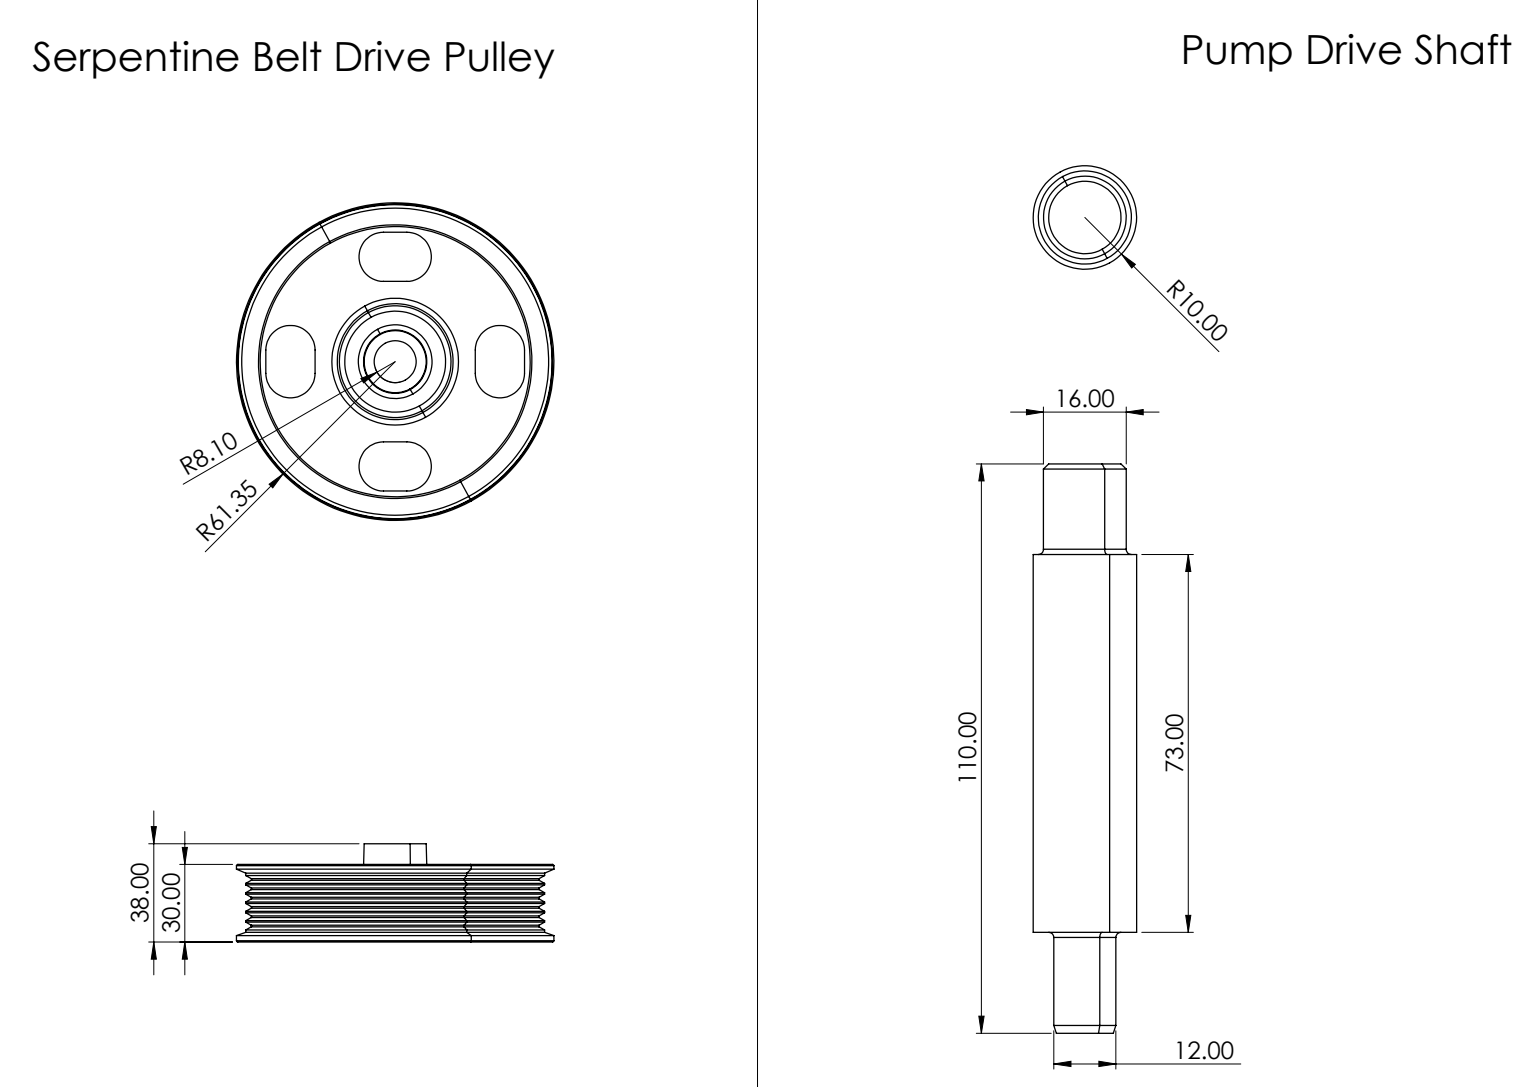
ISO-10303-21;
HEADER;
FILE_DESCRIPTION (('STEP AP214'),
    '1' );
FILE_NAME ('Serpentine Belt Drive Pulley.step',
    '2026-10-09T13:19:41',
    ( '' ),
    ( '' ),
    'SwSTEP 2.0',
    'SolidWorks 2026',
    '' );
FILE_SCHEMA (( 'AUTOMOTIVE_DESIGN' ));
ENDSEC;

DATA;
#8=CARTESIAN_POINT ( 'NONE',  ( 11.78548194719999920, -15.31994771319999948, 21.57317999869999881 ) ) ;
#14=CARTESIAN_POINT ( 'NONE',  ( 0.000000000000000000, -31.69999999999999929, 0.000000000000000000 ) ) ;
#18=CIRCLE ( 'NONE', #19870, 0.3500000000000003664 ) ;
#20=ORIENTED_EDGE ( 'NONE', *, *, #20137, .T. ) ;
#22=VERTEX_POINT ( 'NONE', #6246 ) ;
#29=DIRECTION ( 'NONE',  ( 0.000000000000000000, -1.000000000000000000, 0.000000000000000000 ) ) ;
#31=DIRECTION ( 'NONE',  ( 0.4794255386042040601, 0.000000000000000000, 0.8775825618903720926 ) ) ;
#44=CONICAL_SURFACE ( 'NONE', #19544, 55.67692378859999280, 1.047197551199999799 ) ;
#54=VERTEX_POINT ( 'NONE', #28244 ) ;
#64=CIRCLE ( 'NONE', #16341, 0.3500000000000003664 ) ;
#76=DIRECTION ( 'NONE',  ( 0.4794255386042042266, 0.000000000000000000, 0.8775825618903720926 ) ) ;
#77=VERTEX_POINT ( 'NONE', #6989 ) ;
#84=DIRECTION ( 'NONE',  ( 1.000000000000000000, 0.000000000000000000, 0.000000000000000000 ) ) ;
#87=VERTEX_POINT ( 'NONE', #24762 ) ;
#100=CIRCLE ( 'NONE', #13575, 52.20000000000000284 ) ;
#103=VERTEX_POINT ( 'NONE', #2623 ) ;
#125=ADVANCED_FACE ( 'NONE', ( #15853 ), #9081, .F. ) ;
#128=ORIENTED_EDGE ( 'NONE', *, *, #22826, .F. ) ;
#143=AXIS2_PLACEMENT_3D ( 'NONE', #11532, #26560, #20442 ) ;
#152=DIRECTION ( 'NONE',  ( 0.4794255386042040601, 0.000000000000000000, 0.8775825618903720926 ) ) ;
#157=EDGE_CURVE ( 'NONE', #20862, #20652, #26784, .T. ) ;
#162=DIRECTION ( 'NONE',  ( 0.000000000000000000, 1.000000000000000000, 0.000000000000000000 ) ) ;
#165=ADVANCED_FACE ( 'NONE', ( #26356 ), #6385, .F. ) ;
#169=DIRECTION ( 'NONE',  ( 0.000000000000000000, 1.000000000000000000, 0.000000000000000000 ) ) ;
#171=CARTESIAN_POINT ( 'NONE',  ( 0.000000000000000000, -37.50000000000000000, 0.000000000000000000 ) ) ;
#172=ORIENTED_EDGE ( 'NONE', *, *, #20476, .T. ) ;
#174=DIRECTION ( 'NONE',  ( 0.4794255386042042266, 0.000000000000000000, 0.8775825618903720926 ) ) ;
#177=DIRECTION ( 'NONE',  ( 0.000000000000000000, 1.000000000000000000, 0.000000000000000000 ) ) ;
#188=DIRECTION ( 'NONE',  ( 0.4794255386042000078, 0.000000000000000000, 0.8775825618903743131 ) ) ;
#190=ORIENTED_EDGE ( 'NONE', *, *, #2721, .F. ) ;
#193=CARTESIAN_POINT ( 'NONE',  ( 0.000000000000000000, -23.00000000000000000, 0.000000000000000000 ) ) ;
#207=AXIS2_PLACEMENT_3D ( 'NONE', #10252, #6026, #27775 ) ;
#218=FACE_OUTER_BOUND ( 'NONE', #16317, .T. ) ;
#231=CYLINDRICAL_SURFACE ( 'NONE', #19067, 8.099999999999997868 ) ;
#245=CIRCLE ( 'NONE', #4394, 58.54999999999999716 ) ;
#250=CIRCLE ( 'NONE', #27231, 57.75000000000000000 ) ;
#255=ADVANCED_FACE ( 'NONE', ( #17790 ), #18406, .F. ) ;
#258=VERTEX_POINT ( 'NONE', #22459 ) ;
#265=CARTESIAN_POINT ( 'NONE',  ( 0.000000000000000000, -26.90310889129999694, 0.000000000000000000 ) ) ;
#268=LINE ( 'NONE', #1996, #17176 ) ;
#307=DIRECTION ( 'NONE',  ( 0.000000000000000000, 1.000000000000000000, 0.000000000000000000 ) ) ;
#316=AXIS2_PLACEMENT_3D ( 'NONE', #22770, #793, #16190 ) ;
#318=CARTESIAN_POINT ( 'NONE',  ( 0.000000000000000000, -11.00000000000000000, 0.000000000000000000 ) ) ;
#352=EDGE_CURVE ( 'NONE', #18033, #14401, #4448, .T. ) ;
#357=EDGE_CURVE ( 'NONE', #20895, #2845, #5405, .T. ) ;
#360=ORIENTED_EDGE ( 'NONE', *, *, #15898, .T. ) ;
#367=AXIS2_PLACEMENT_3D ( 'NONE', #6686, #4637, #15550 ) ;
#368=ADVANCED_FACE ( 'NONE', ( #27069 ), #19745, .T. ) ;
#369=CIRCLE ( 'NONE', #15692, 60.85000000000000142 ) ;
#370=DIRECTION ( 'NONE',  ( 0.000000000000000000, 1.000000000000000000, 0.000000000000000000 ) ) ;
#384=CARTESIAN_POINT ( 'NONE',  ( 3.883346862689999845, -2.000000000000000000, 7.108418751309999450 ) ) ;
#385=AXIS2_PLACEMENT_3D ( 'NONE', #10663, #12718, #21630 ) ;
#398=AXIS2_PLACEMENT_3D ( 'NONE', #25664, #5557, #14574 ) ;
#408=DIRECTION ( 'NONE',  ( 0.000000000000000000, 1.000000000000000000, 0.000000000000000000 ) ) ;
#412=CIRCLE ( 'NONE', #28280, 57.75000000000000000 ) ;
#422=ORIENTED_EDGE ( 'NONE', *, *, #27436, .F. ) ;
#424=CARTESIAN_POINT ( 'NONE',  ( -4.500000000000000000, -11.00000000000000000, 31.00000000000000000 ) ) ;
#429=EDGE_CURVE ( 'NONE', #15620, #8975, #245, .T. ) ;
#432=DIRECTION ( 'NONE',  ( -1.000000000000000000, 0.000000000000000000, -4.565061778886334044E-16 ) ) ;
#433=DIRECTION ( 'NONE',  ( 0.4151946956541399669, 0.5000000000001689759, 0.7600087925152558821 ) ) ;
#436=DIRECTION ( 'NONE',  ( -1.224606353819999829E-16, 0.000000000000000000, 1.000000000000000000 ) ) ;
#454=CONICAL_SURFACE ( 'NONE', #1820, 55.67692378859999280, 1.047197551199999799 ) ;
#456=EDGE_CURVE ( 'NONE', #25924, #731, #15538, .T. ) ;
#459=CARTESIAN_POINT ( 'NONE',  ( 27.68682485439999752, -17.30000000000000071, 50.68039294919999804 ) ) ;
#463=DIRECTION ( 'NONE',  ( 0.000000000000000000, 1.000000000000000000, 0.000000000000000000 ) ) ;
#467=ADVANCED_FACE ( 'NONE', ( #20064 ), #15828, .T. ) ;
#474=DIRECTION ( 'NONE',  ( 0.000000000000000000, 1.000000000000000000, 0.000000000000000000 ) ) ;
#476=EDGE_LOOP ( 'NONE', ( #14422, #15237, #5808, #25954 ) ) ;
#481=DIRECTION ( 'NONE',  ( 0.000000000000000000, 1.000000000000000000, 0.000000000000000000 ) ) ;
#484=ORIENTED_EDGE ( 'NONE', *, *, #2417, .F. ) ;
#490=DIRECTION ( 'NONE',  ( 0.4794255386042036715, 0.000000000000000000, 0.8775825618903724257 ) ) ;
#503=EDGE_CURVE ( 'NONE', #1478, #12804, #17430, .T. ) ;
#509=EDGE_LOOP ( 'NONE', ( #14292, #25818, #23874, #1797 ) ) ;
#513=FACE_OUTER_BOUND ( 'NONE', #18198, .T. ) ;
#519=VERTEX_POINT ( 'NONE', #424 ) ;
#526=CARTESIAN_POINT ( 'NONE',  ( 5.873292863139999653, -11.55246854740000018, 10.75099047199999980 ) ) ;
#530=FACE_OUTER_BOUND ( 'NONE', #1949, .T. ) ;
#546=CARTESIAN_POINT ( 'NONE',  ( 27.68682485439999752, -14.30000000000000071, 50.68039294919999804 ) ) ;
#550=ORIENTED_EDGE ( 'NONE', *, *, #21053, .T. ) ;
#575=DIRECTION ( 'NONE',  ( 0.4794255386042000078, 0.000000000000000000, 0.8775825618903743131 ) ) ;
#577=VECTOR ( 'NONE', #18094, 1000.000000000000000 ) ;
#579=VECTOR ( 'NONE', #5626, 999.9999999999998863 ) ;
#581=CARTESIAN_POINT ( 'NONE',  ( 0.000000000000000000, -37.08699221940000257, 0.000000000000000000 ) ) ;
#584=VERTEX_POINT ( 'NONE', #13793 ) ;
#594=ORIENTED_EDGE ( 'NONE', *, *, #7560, .T. ) ;
#599=ORIENTED_EDGE ( 'NONE', *, *, #25882, .T. ) ;
#604=ORIENTED_EDGE ( 'NONE', *, *, #24072, .T. ) ;
#618=VERTEX_POINT ( 'NONE', #23274 ) ;
#636=ORIENTED_EDGE ( 'NONE', *, *, #17902, .T. ) ;
#640=VERTEX_POINT ( 'NONE', #18620 ) ;
#669=EDGE_CURVE ( 'NONE', #15395, #12657, #1152, .T. ) ;
#673=EDGE_CURVE ( 'NONE', #12096, #23467, #9990, .T. ) ;
#691=CIRCLE ( 'NONE', #4371, 24.76278252470000041 ) ;
#703=DIRECTION ( 'NONE',  ( 0.000000000000000000, 1.000000000000000000, 0.000000000000000000 ) ) ;
#704=TOROIDAL_SURFACE ( 'NONE', #18826, 25.11294200180000047, 0.5000000000000000000 ) ;
#721=LINE ( 'NONE', #9422, #6410 ) ;
#731=VERTEX_POINT ( 'NONE', #1559 ) ;
#736=CIRCLE ( 'NONE', #10888, 0.3500000000000003664 ) ;
#739=AXIS2_PLACEMENT_3D ( 'NONE', #22838, #3037, #27350 ) ;
#764=ORIENTED_EDGE ( 'NONE', *, *, #15472, .F. ) ;
#765=CARTESIAN_POINT ( 'NONE',  ( 25.57735248450000043, -16.00000000000000000, 46.81902967690000139 ) ) ;
#770=ORIENTED_EDGE ( 'NONE', *, *, #5118, .F. ) ;
#786=CIRCLE ( 'NONE', #28633, 0.3500000000000003664 ) ;
#793=DIRECTION ( 'NONE',  ( 0.000000000000000000, 1.000000000000000000, 0.000000000000000000 ) ) ;
#803=VECTOR ( 'NONE', #16768, 999.9999999999998863 ) ;
#810=DIRECTION ( 'NONE',  ( 1.000000000000000000, 0.000000000000000000, 0.000000000000000000 ) ) ;
#852=ORIENTED_EDGE ( 'NONE', *, *, #4107, .F. ) ;
#859=CIRCLE ( 'NONE', #18511, 57.75000000000000000 ) ;
#863=CARTESIAN_POINT ( 'NONE',  ( 4.500000000000000000, -13.00000000000000000, -50.00000000000000000 ) ) ;
#872=DIRECTION ( 'NONE',  ( 0.000000000000000000, 0.000000000000000000, -1.000000000000000000 ) ) ;
#900=CIRCLE ( 'NONE', #15733, 53.35000000000000142 ) ;
#914=VERTEX_POINT ( 'NONE', #15022 ) ;
#940=AXIS2_PLACEMENT_3D ( 'NONE', #13156, #4429, #22204 ) ;
#943=ADVANCED_FACE ( 'NONE', ( #22484 ), #23059, .T. ) ;
#954=CARTESIAN_POINT ( 'NONE',  ( 0.000000000000000000, -10.00000000000000000, 60.66666666670000296 ) ) ;
#963=DIRECTION ( 'NONE',  ( 0.3422283636740854340, 0.7003189540771749266, 0.6264448177271558782 ) ) ;
#975=ORIENTED_EDGE ( 'NONE', *, *, #2781, .F. ) ;
#984=AXIS2_PLACEMENT_3D ( 'NONE', #22104, #28780, #24280 ) ;
#999=FACE_OUTER_BOUND ( 'NONE', #16209, .T. ) ;
#1007=LINE ( 'NONE', #25323, #579 ) ;
#1009=ORIENTED_EDGE ( 'NONE', *, *, #8094, .T. ) ;
#1033=CARTESIAN_POINT ( 'NONE',  ( 0.000000000000000000, -2.000000000000000000, 0.000000000000000000 ) ) ;
#1048=TOROIDAL_SURFACE ( 'NONE', #18699, 57.54999999999999716, 1.000000000000000000 ) ;
#1057=ORIENTED_EDGE ( 'NONE', *, *, #2655, .F. ) ;
#1060=CIRCLE ( 'NONE', #4744, 14.25000000000000000 ) ;
#1067=ORIENTED_EDGE ( 'NONE', *, *, #7433, .T. ) ;
#1075=ORIENTED_EDGE ( 'NONE', *, *, #3374, .F. ) ;
#1104=AXIS2_PLACEMENT_3D ( 'NONE', #1320, #19082, #16896 ) ;
#1110=DIRECTION ( 'NONE',  ( 0.000000000000000000, -1.000000000000000000, 0.000000000000000000 ) ) ;
#1114=CARTESIAN_POINT ( 'NONE',  ( 0.000000000000000000, -15.14308496720000008, 0.000000000000000000 ) ) ;
#1122=CONICAL_SURFACE ( 'NONE', #9854, 11.99999999999999822, 0.02623728384790100648 ) ;
#1131=CYLINDRICAL_SURFACE ( 'NONE', #24779, 61.34999999999998721 ) ;
#1132=ORIENTED_EDGE ( 'NONE', *, *, #23898, .T. ) ;
#1134=ADVANCED_FACE ( 'NONE', ( #21028 ), #16056, .T. ) ;
#1142=CARTESIAN_POINT ( 'NONE',  ( 0.000000000000000000, -2.000000000000000000, 0.000000000000000000 ) ) ;
#1145=DIRECTION ( 'NONE',  ( 1.000000000000000000, 0.000000000000000000, 0.000000000000000000 ) ) ;
#1150=CONICAL_SURFACE ( 'NONE', #12714, 21.60095686220001454, 0.7949521073230001456 ) ;
#1152=LINE ( 'NONE', #7700, #5344 ) ;
#1170=ORIENTED_EDGE ( 'NONE', *, *, #26606, .F. ) ;
#1174=CARTESIAN_POINT ( 'NONE',  ( 0.000000000000000000, -17.50000000000000000, 9.099999999999999645 ) ) ;
#1180=DIRECTION ( 'NONE',  ( 1.000000000000000000, 0.000000000000000000, 0.000000000000000000 ) ) ;
#1181=VERTEX_POINT ( 'NONE', #28133 ) ;
#1186=EDGE_CURVE ( 'NONE', #5075, #17731, #27244, .T. ) ;
#1194=EDGE_LOOP ( 'NONE', ( #8651, #2603, #6295, #28164 ) ) ;
#1196=EDGE_CURVE ( 'NONE', #14426, #19773, #20727, .T. ) ;
#1201=ORIENTED_EDGE ( 'NONE', *, *, #3911, .F. ) ;
#1212=FACE_OUTER_BOUND ( 'NONE', #25199, .T. ) ;
#1222=EDGE_CURVE ( 'NONE', #14011, #25949, #25369, .T. ) ;
#1223=DIRECTION ( 'NONE',  ( 1.000000000000000000, 0.000000000000000000, 0.000000000000000000 ) ) ;
#1228=CARTESIAN_POINT ( 'NONE',  ( 0.000000000000000000, -36.20000000000000284, 0.000000000000000000 ) ) ;
#1234=VERTEX_POINT ( 'NONE', #26969 ) ;
#1239=DIRECTION ( 'NONE',  ( 0.4794255386042000078, 0.000000000000000000, 0.8775825618903743131 ) ) ;
#1252=DIRECTION ( 'NONE',  ( 0.4794255386042040601, 0.000000000000000000, 0.8775825618903720926 ) ) ;
#1258=CARTESIAN_POINT ( 'NONE',  ( -4.500000000000000000, -15.00000000000000000, 40.50000000000000000 ) ) ;
#1269=DIRECTION ( 'NONE',  ( 1.000000000000000000, 0.000000000000000000, 0.000000000000000000 ) ) ;
#1274=ORIENTED_EDGE ( 'NONE', *, *, #6243, .T. ) ;
#1286=DIRECTION ( 'NONE',  ( -1.000000000000000000, 0.000000000000000000, 0.000000000000000000 ) ) ;
#1299=CIRCLE ( 'NONE', #22695, 52.86371681420000357 ) ;
#1320=CARTESIAN_POINT ( 'NONE',  ( 0.000000000000000000, -2.000000000000000000, 8.099999999999999645 ) ) ;
#1323=AXIS2_PLACEMENT_3D ( 'NONE', #7852, #12345, #17150 ) ;
#1336=EDGE_LOOP ( 'NONE', ( #27422, #1067, #8213, #19531 ) ) ;
#1337=CIRCLE ( 'NONE', #5040, 55.67692378859999991 ) ;
#1338=FACE_OUTER_BOUND ( 'NONE', #23635, .T. ) ;
#1339=AXIS2_PLACEMENT_3D ( 'NONE', #8246, #19612, #25892 ) ;
#1348=CARTESIAN_POINT ( 'NONE',  ( 28.07036528529999941, -39.32601556110000018, 51.38245899869999533 ) ) ;
#1357=ORIENTED_EDGE ( 'NONE', *, *, #15472, .T. ) ;
#1360=DIRECTION ( 'NONE',  ( 0.000000000000000000, -1.000000000000000000, 0.000000000000000000 ) ) ;
#1369=CARTESIAN_POINT ( 'NONE',  ( -31.00000000000000000, 0.000000000000000000, -4.500000000000000000 ) ) ;
#1373=AXIS2_PLACEMENT_3D ( 'NONE', #19047, #27930, #7968 ) ;
#1377=EDGE_CURVE ( 'NONE', #2012, #20039, #5529, .T. ) ;
#1381=EDGE_CURVE ( 'NONE', #22328, #8830, #3355, .T. ) ;
#1383=TOROIDAL_SURFACE ( 'NONE', #5566, 14.25000000000000000, 2.000000000000000000 ) ;
#1386=AXIS2_PLACEMENT_3D ( 'NONE', #5883, #3432, #1535 ) ;
#1392=( LENGTH_UNIT ( ) NAMED_UNIT ( * ) SI_UNIT ( .MILLI., .METRE. ) );
#1394=AXIS2_PLACEMENT_3D ( 'NONE', #27280, #26988, #18533 ) ;
#1401=CIRCLE ( 'NONE', #5114, 61.35000000000000142 ) ;
#1412=EDGE_LOOP ( 'NONE', ( #2757, #20982, #9366, #23861 ) ) ;
#1424=ORIENTED_EDGE ( 'NONE', *, *, #18031, .F. ) ;
#1434=ADVANCED_FACE ( 'NONE', ( #8401 ), #24419, .F. ) ;
#1441=DIRECTION ( 'NONE',  ( 0.000000000000000000, 1.000000000000000000, 0.000000000000000000 ) ) ;
#1449=ORIENTED_EDGE ( 'NONE', *, *, #5830, .T. ) ;
#1451=CIRCLE ( 'NONE', #4700, 0.4999999999999981126 ) ;
#1454=ORIENTED_EDGE ( 'NONE', *, *, #12507, .T. ) ;
#1456=CARTESIAN_POINT ( 'NONE',  ( 31.00000000000000000, -11.00000000000000000, 1.953992523340000041E-14 ) ) ;
#1457=ORIENTED_EDGE ( 'NONE', *, *, #19024, .T. ) ;
#1478=VERTEX_POINT ( 'NONE', #27890 ) ;
#1494=CARTESIAN_POINT ( 'NONE',  ( 0.000000000000000000, -40.00000000000000000, 60.85000000000000142 ) ) ;
#1497=CONICAL_SURFACE ( 'NONE', #22909, 57.74999999999999289, 1.152571997220000144 ) ;
#1519=VECTOR ( 'NONE', #12148, 1000.000000000000000 ) ;
#1535=DIRECTION ( 'NONE',  ( 0.4794255386042040601, 0.000000000000000000, 0.8775825618903720926 ) ) ;
#1536=EDGE_LOOP ( 'NONE', ( #13375, #8343, #24939, #21800 ) ) ;
#1559=CARTESIAN_POINT ( 'NONE',  ( 26.69293917519999937, -22.69689110870000093, 48.86109741659999628 ) ) ;
#1563=DIRECTION ( 'NONE',  ( 0.000000000000000000, -1.000000000000000000, 0.000000000000000000 ) ) ;
#1567=CIRCLE ( 'NONE', #15021, 60.66666666670000296 ) ;
#1595=EDGE_LOOP ( 'NONE', ( #10372, #9875, #25781, #7720 ) ) ;
#1599=EDGE_LOOP ( 'NONE', ( #20525, #22685, #3053, #14488 ) ) ;
#1610=CARTESIAN_POINT ( 'NONE',  ( -27.68682485439999752, -32.30000000000000426, -50.68039294919999804 ) ) ;
#1618=AXIS2_PLACEMENT_3D ( 'NONE', #8826, #2740, #575 ) ;
#1621=CARTESIAN_POINT ( 'NONE',  ( 0.000000000000000000, -33.49689110869999809, 0.000000000000000000 ) ) ;
#1637=FACE_OUTER_BOUND ( 'NONE', #11830, .T. ) ;
#1640=DIRECTION ( 'NONE',  ( 1.000000000000000000, 0.000000000000000000, 0.000000000000000000 ) ) ;
#1649=CIRCLE ( 'NONE', #16987, 0.3500000000000003664 ) ;
#1654=ORIENTED_EDGE ( 'NONE', *, *, #12704, .T. ) ;
#1656=EDGE_CURVE ( 'NONE', #15453, #19773, #6655, .T. ) ;
#1668=EDGE_LOOP ( 'NONE', ( #8051, #17208, #12347, #594 ) ) ;
#1699=CARTESIAN_POINT ( 'NONE',  ( -9.348798002780000616, -17.50000000000000000, -17.11285995690000306 ) ) ;
#1704=CARTESIAN_POINT ( 'NONE',  ( 0.000000000000000000, -11.79999999999999893, 0.000000000000000000 ) ) ;
#1711=DIRECTION ( 'NONE',  ( 1.000000000000000000, 0.000000000000000000, 0.000000000000000000 ) ) ;
#1732=CARTESIAN_POINT ( 'NONE',  ( 0.000000000000000000, -11.00000000000000000, 0.000000000000000000 ) ) ;
#1737=ORIENTED_EDGE ( 'NONE', *, *, #10273, .F. ) ;
#1742=CIRCLE ( 'NONE', #25487, 24.40223267850000255 ) ;
#1746=EDGE_CURVE ( 'NONE', #914, #1181, #8053, .T. ) ;
#1750=DIRECTION ( 'NONE',  ( 0.4794255386042040046, 0.000000000000000000, 0.8775825618903722036 ) ) ;
#1752=DIRECTION ( 'NONE',  ( 0.4794255386042059475, 0.000000000000000000, 0.8775825618903710934 ) ) ;
#1753=EDGE_CURVE ( 'NONE', #8830, #25924, #27612, .T. ) ;
#1757=ORIENTED_EDGE ( 'NONE', *, *, #22845, .T. ) ;
#1760=ORIENTED_EDGE ( 'NONE', *, *, #23659, .T. ) ;
#1766=DIRECTION ( 'NONE',  ( 0.4794255386042040046, 0.000000000000000000, 0.8775825618903720926 ) ) ;
#1768=DIRECTION ( 'NONE',  ( 0.4794255386042000078, 0.000000000000000000, 0.8775825618903743131 ) ) ;
#1769=DIRECTION ( 'NONE',  ( 0.000000000000000000, 1.000000000000000000, 0.000000000000000000 ) ) ;
#1773=VECTOR ( 'NONE', #7996, 1000.000000000000000 ) ;
#1786=( GEOMETRIC_REPRESENTATION_CONTEXT ( 3 ) GLOBAL_UNCERTAINTY_ASSIGNED_CONTEXT ( ( #20546 ) ) GLOBAL_UNIT_ASSIGNED_CONTEXT ( ( #25669, #21288, #14718 ) ) REPRESENTATION_CONTEXT ( 'NONE', 'WORKASPACE' ) );
#1797=ORIENTED_EDGE ( 'NONE', *, *, #15743, .F. ) ;
#1801=CARTESIAN_POINT ( 'NONE',  ( -25.02601311510000315, -11.00000000000000000, -45.80980973070000317 ) ) ;
#1802=ORIENTED_EDGE ( 'NONE', *, *, #26480, .T. ) ;
#1819=AXIS2_PLACEMENT_3D ( 'NONE', #7307, #9621, #5264 ) ;
#1820=AXIS2_PLACEMENT_3D ( 'NONE', #12023, #27649, #7692 ) ;
#1834=AXIS2_PLACEMENT_3D ( 'NONE', #19061, #20420, #490 ) ;
#1840=ADVANCED_FACE ( 'NONE', ( #6565 ), #11765, .T. ) ;
#1843=CARTESIAN_POINT ( 'NONE',  ( -29.08514934200000113, -20.00000000000000000, -53.24000875469999983 ) ) ;
#1846=CYLINDRICAL_SURFACE ( 'NONE', #7110, 57.74999999999999289 ) ;
#1856=VERTEX_POINT ( 'NONE', #10899 ) ;
#1868=CARTESIAN_POINT ( 'NONE',  ( -29.41275679339999982, -25.00000000000000000, -53.83969017199999740 ) ) ;
#1871=VERTEX_POINT ( 'NONE', #26828 ) ;
#1874=ORIENTED_EDGE ( 'NONE', *, *, #16751, .T. ) ;
#1875=EDGE_CURVE ( 'NONE', #1478, #12096, #8721, .T. ) ;
#1900=AXIS2_PLACEMENT_3D ( 'NONE', #27713, #25243, #5270 ) ;
#1914=ORIENTED_EDGE ( 'NONE', *, *, #6174, .F. ) ;
#1929=ORIENTED_EDGE ( 'NONE', *, *, #4004, .F. ) ;
#1930=LINE ( 'NONE', #19682, #6678 ) ;
#1933=ORIENTED_EDGE ( 'NONE', *, *, #10541, .T. ) ;
#1944=VERTEX_POINT ( 'NONE', #26975 ) ;
#1945=DIRECTION ( 'NONE',  ( 0.000000000000000000, 1.000000000000000000, 0.000000000000000000 ) ) ;
#1947=EDGE_CURVE ( 'NONE', #19954, #26186, #16169, .T. ) ;
#1949=EDGE_LOOP ( 'NONE', ( #6217, #17280, #3392, #19503 ) ) ;
#1957=ORIENTED_EDGE ( 'NONE', *, *, #7433, .F. ) ;
#1965=DIRECTION ( 'NONE',  ( 0.000000000000000000, 1.000000000000000000, 0.000000000000000000 ) ) ;
#1976=ORIENTED_EDGE ( 'NONE', *, *, #15304, .F. ) ;
#1985=DIRECTION ( 'NONE',  ( 0.000000000000000000, 1.000000000000000000, 0.000000000000000000 ) ) ;
#1988=ORIENTED_EDGE ( 'NONE', *, *, #18804, .T. ) ;
#1992=DIRECTION ( 'NONE',  ( 1.000000000000000000, 0.000000000000000000, 0.000000000000000000 ) ) ;
#1994=DIRECTION ( 'NONE',  ( 0.000000000000000000, 0.000000000000000000, 1.000000000000000000 ) ) ;
#1996=CARTESIAN_POINT ( 'NONE',  ( 27.18988201479999844, -31.10155444569999617, 49.77074518290000071 ) ) ;
#2002=AXIS2_PLACEMENT_3D ( 'NONE', #16319, #2648, #20557 ) ;
#2005=VECTOR ( 'NONE', #1563, 1000.000000000000000 ) ;
#2012=VERTEX_POINT ( 'NONE', #7159 ) ;
#2023=AXIS2_PLACEMENT_3D ( 'NONE', #12263, #20751, #18979 ) ;
#2026=ORIENTED_EDGE ( 'NONE', *, *, #15396, .F. ) ;
#2033=CARTESIAN_POINT ( 'NONE',  ( -9.348798002780000616, -13.50000000000000000, -17.11285995690000306 ) ) ;
#2039=VERTEX_POINT ( 'NONE', #2791 ) ;
#2041=DIRECTION ( 'NONE',  ( 0.4794255386042036715, 0.000000000000000000, 0.8775825618903724257 ) ) ;
#2042=CARTESIAN_POINT ( 'NONE',  ( 0.000000000000000000, -17.50000000000000000, 0.000000000000000000 ) ) ;
#2050=EDGE_CURVE ( 'NONE', #2986, #9393, #22604, .T. ) ;
#2052=VECTOR ( 'NONE', #28538, 1000.000000000000114 ) ;
#2058=ORIENTED_EDGE ( 'NONE', *, *, #21512, .F. ) ;
#2068=DIRECTION ( 'NONE',  ( 0.4794255386042040601, 0.000000000000000000, 0.8775825618903720926 ) ) ;
#2085=ADVANCED_FACE ( 'NONE', ( #25503 ), #5278, .F. ) ;
#2087=ORIENTED_EDGE ( 'NONE', *, *, #429, .T. ) ;
#2100=DIRECTION ( 'NONE',  ( 0.000000000000000000, 1.000000000000000000, 0.000000000000000000 ) ) ;
#2115=DIRECTION ( 'NONE',  ( 0.000000000000000000, 1.000000000000000000, 0.000000000000000000 ) ) ;
#2118=DIRECTION ( 'NONE',  ( 0.4794255386042041156, 0.000000000000000000, 0.8775825618903722036 ) ) ;
#2134=DIRECTION ( 'NONE',  ( 0.4794255386042040601, 0.000000000000000000, 0.8775825618903720926 ) ) ;
#2137=CIRCLE ( 'NONE', #22635, 52.86371681420000357 ) ;
#2138=PLANE ( 'NONE',  #18692 ) ;
#2150=DIRECTION ( 'NONE',  ( 0.4794255386042036715, 0.000000000000000000, 0.8775825618903724257 ) ) ;
#2153=VERTEX_POINT ( 'NONE', #27966 ) ;
#2154=ADVANCED_FACE ( 'NONE', ( #23872, #16748 ), #8005, .T. ) ;
#2165=ORIENTED_EDGE ( 'NONE', *, *, #16459, .T. ) ;
#2190=CARTESIAN_POINT ( 'NONE',  ( 0.000000000000000000, -14.00000000000000000, 0.000000000000000000 ) ) ;
#2194=DIRECTION ( 'NONE',  ( 0.000000000000000000, 1.000000000000000000, 0.000000000000000000 ) ) ;
#2195=ORIENTED_EDGE ( 'NONE', *, *, #16351, .F. ) ;
#2197=EDGE_CURVE ( 'NONE', #19419, #16942, #10351, .T. ) ;
#2216=DIRECTION ( 'NONE',  ( -0.8775825618903722036, 0.000000000000000000, 0.4794255386042041156 ) ) ;
#2223=CIRCLE ( 'NONE', #14769, 58.54999999999999716 ) ;
#2226=CYLINDRICAL_SURFACE ( 'NONE', #28044, 57.74999999999999289 ) ;
#2240=ADVANCED_FACE ( 'NONE', ( #15238 ), #26346, .T. ) ;
#2241=CARTESIAN_POINT ( 'NONE',  ( 0.000000000000000000, -20.89999999999999858, 0.000000000000000000 ) ) ;
#2252=PRODUCT ( 'Serpentine Belt Drive Pulley', 'Serpentine Belt Drive Pulley', '', ( #8864 ) ) ;
#2256=CARTESIAN_POINT ( 'NONE',  ( 0.000000000000000000, -20.00000000000000000, 0.000000000000000000 ) ) ;
#2258=VERTEX_POINT ( 'NONE', #24299 ) ;
#2260=VECTOR ( 'NONE', #22969, 999.9999999999998863 ) ;
#2275=CARTESIAN_POINT ( 'NONE',  ( 0.000000000000000000, -16.50000000000000000, 0.000000000000000000 ) ) ;
#2280=AXIS2_PLACEMENT_3D ( 'NONE', #3506, #12364, #16326 ) ;
#2282=FACE_OUTER_BOUND ( 'NONE', #10560, .T. ) ;
#2295=CIRCLE ( 'NONE', #13919, 9.500000000000000000 ) ;
#2299=CIRCLE ( 'NONE', #5564, 57.75000000000000000 ) ;
#2330=FACE_OUTER_BOUND ( 'NONE', #5988, .T. ) ;
#2339=EDGE_LOOP ( 'NONE', ( #24017, #18856, #23774, #28014 ) ) ;
#2342=ORIENTED_EDGE ( 'NONE', *, *, #23406, .F. ) ;
#2345=CARTESIAN_POINT ( 'NONE',  ( 2.220446049249999745E-14, -15.00000000000000000, -50.00000000000000000 ) ) ;
#2347=ADVANCED_FACE ( 'NONE', ( #11160 ), #18185, .T. ) ;
#2355=FACE_OUTER_BOUND ( 'NONE', #19327, .T. ) ;
#2359=AXIS2_PLACEMENT_3D ( 'NONE', #13477, #22829, #2870 ) ;
#2364=CIRCLE ( 'NONE', #21427, 57.75000000000000000 ) ;
#2371=EDGE_CURVE ( 'NONE', #6736, #4998, #4926, .T. ) ;
#2377=CARTESIAN_POINT ( 'NONE',  ( -26.69293917519999937, -19.09689110869999951, -48.86109741659999628 ) ) ;
#2383=TOROIDAL_SURFACE ( 'NONE', #10709, 55.85192378860000417, 0.3499999999999999778 ) ;
#2384=CIRCLE ( 'NONE', #27960, 55.67692378859999991 ) ;
#2389=VECTOR ( 'NONE', #15810, 1000.000000000000000 ) ;
#2396=CARTESIAN_POINT ( 'NONE',  ( 0.000000000000000000, -23.00000000000000000, 0.000000000000000000 ) ) ;
#2398=DIRECTION ( 'NONE',  ( 0.000000000000000000, 1.000000000000000000, 0.000000000000000000 ) ) ;
#2412=EDGE_CURVE ( 'NONE', #19945, #16942, #21521, .T. ) ;
#2416=FACE_OUTER_BOUND ( 'NONE', #12610, .T. ) ;
#2417=EDGE_CURVE ( 'NONE', #8384, #18741, #27081, .T. ) ;
#2427=ORIENTED_EDGE ( 'NONE', *, *, #12208, .T. ) ;
#2431=DIRECTION ( 'NONE',  ( 0.4751828347227322613, 0.1327433628319252545, 0.8698163445285104212 ) ) ;
#2434=FACE_OUTER_BOUND ( 'NONE', #10940, .T. ) ;
#2457=ADVANCED_FACE ( 'NONE', ( #3186 ), #1122, .T. ) ;
#2464=CARTESIAN_POINT ( 'NONE',  ( 31.00000000000000000, 0.000000000000000000, 4.500000000000000000 ) ) ;
#2487=DIRECTION ( 'NONE',  ( 0.4794255386042040601, 0.000000000000000000, 0.8775825618903720926 ) ) ;
#2490=CIRCLE ( 'NONE', #13571, 61.35000000000000142 ) ;
#2491=AXIS2_PLACEMENT_3D ( 'NONE', #18706, #27860, #8044 ) ;
#2498=ORIENTED_EDGE ( 'NONE', *, *, #27253, .T. ) ;
#2506=EDGE_LOOP ( 'NONE', ( #7714, #6725, #4166, #19968 ) ) ;
#2520=CARTESIAN_POINT ( 'NONE',  ( 0.000000000000000000, -10.50000000000000000, 0.000000000000000000 ) ) ;
#2528=EDGE_CURVE ( 'NONE', #11029, #12945, #19681, .T. ) ;
#2557=PLANE ( 'NONE',  #24883 ) ;
#2560=DIRECTION ( 'NONE',  ( 0.000000000000000000, 1.000000000000000000, 0.000000000000000000 ) ) ;
#2565=CARTESIAN_POINT ( 'NONE',  ( 0.000000000000000000, -20.89999999999999858, 0.000000000000000000 ) ) ;
#2573=ORIENTED_EDGE ( 'NONE', *, *, #17303, .T. ) ;
#2577=EDGE_LOOP ( 'NONE', ( #9350, #10710, #7557, #28137 ) ) ;
#2580=CYLINDRICAL_SURFACE ( 'NONE', #13699, 9.500000000000001776 ) ;
#2590=ORIENTED_EDGE ( 'NONE', *, *, #6883, .T. ) ;
#2599=ORIENTED_EDGE ( 'NONE', *, *, #20782, .F. ) ;
#2603=ORIENTED_EDGE ( 'NONE', *, *, #23973, .T. ) ;
#2609=ORIENTED_EDGE ( 'NONE', *, *, #6058, .F. ) ;
#2623=CARTESIAN_POINT ( 'NONE',  ( -27.68682485439999752, -14.30000000000000071, -50.68039294919999804 ) ) ;
#2625=EDGE_CURVE ( 'NONE', #7539, #5596, #14520, .T. ) ;
#2629=EDGE_CURVE ( 'NONE', #8365, #14272, #16715, .T. ) ;
#2635=ORIENTED_EDGE ( 'NONE', *, *, #22928, .T. ) ;
#2648=DIRECTION ( 'NONE',  ( 0.000000000000000000, 1.000000000000000000, 0.000000000000000000 ) ) ;
#2655=EDGE_CURVE ( 'NONE', #15179, #8526, #2490, .T. ) ;
#2671=DIRECTION ( 'NONE',  ( 0.4794255386042041156, 0.000000000000000000, 0.8775825618903720926 ) ) ;
#2696=AXIS2_PLACEMENT_3D ( 'NONE', #17695, #28613, #4289 ) ;
#2708=DIRECTION ( 'NONE',  ( 0.000000000000000000, 1.000000000000000000, 0.000000000000000000 ) ) ;
#2712=CARTESIAN_POINT ( 'NONE',  ( 27.68682485439999752, -24.80000000000000071, 50.68039294919999804 ) ) ;
#2714=ORIENTED_EDGE ( 'NONE', *, *, #18312, .T. ) ;
#2716=AXIS2_PLACEMENT_3D ( 'NONE', #4651, #13234, #17479 ) ;
#2718=EDGE_LOOP ( 'NONE', ( #27894, #16569, #23075, #22728 ) ) ;
#2721=EDGE_CURVE ( 'NONE', #21247, #17262, #18248, .T. ) ;
#2723=CARTESIAN_POINT ( 'NONE',  ( 0.000000000000000000, -30.20000000000000284, 0.000000000000000000 ) ) ;
#2730=CIRCLE ( 'NONE', #20874, 2.999999999999999556 ) ;
#2740=DIRECTION ( 'NONE',  ( 0.8775825618903722036, 0.000000000000000000, -0.4794255386042041156 ) ) ;
#2746=ORIENTED_EDGE ( 'NONE', *, *, #8123, .T. ) ;
#2748=CARTESIAN_POINT ( 'NONE',  ( 27.18988201479999844, -25.69844555429999744, 49.77074518290000071 ) ) ;
#2750=ORIENTED_EDGE ( 'NONE', *, *, #10665, .T. ) ;
#2753=DIRECTION ( 'NONE',  ( 1.000000000000000000, 0.000000000000000000, 0.000000000000000000 ) ) ;
#2757=ORIENTED_EDGE ( 'NONE', *, *, #18056, .F. ) ;
#2774=CYLINDRICAL_SURFACE ( 'NONE', #25788, 57.74999999999999289 ) ;
#2775=EDGE_LOOP ( 'NONE', ( #20148, #24485, #15477, #18761 ) ) ;
#2780=DIRECTION ( 'NONE',  ( 0.000000000000000000, 1.000000000000000000, 0.000000000000000000 ) ) ;
#2781=EDGE_CURVE ( 'NONE', #731, #6736, #12177, .T. ) ;
#2783=DIRECTION ( 'NONE',  ( 0.000000000000000000, 1.000000000000000000, 0.000000000000000000 ) ) ;
#2784=DIRECTION ( 'NONE',  ( -0.4509255599460827435, -0.3396444637780623443, -0.8254137008871517134 ) ) ;
#2791=CARTESIAN_POINT ( 'NONE',  ( -26.69293917519999937, -15.49689110870000164, -48.86109741659999628 ) ) ;
#2806=DIRECTION ( 'NONE',  ( 1.000000000000000000, 0.000000000000000000, 0.000000000000000000 ) ) ;
#2813=FACE_OUTER_BOUND ( 'NONE', #11451, .T. ) ;
#2816=ADVANCED_FACE ( 'NONE', ( #6344 ), #1846, .T. ) ;
#2826=CARTESIAN_POINT ( 'NONE',  ( 4.500000000000000000, -11.00000000000000000, 31.00000000000000000 ) ) ;
#2845=VERTEX_POINT ( 'NONE', #6494 ) ;
#2858=CARTESIAN_POINT ( 'NONE',  ( 0.000000000000000000, -37.08699221940000257, 0.000000000000000000 ) ) ;
#2861=DIRECTION ( 'NONE',  ( 0.000000000000000000, -1.000000000000000000, 0.000000000000000000 ) ) ;
#2863=ORIENTED_EDGE ( 'NONE', *, *, #21763, .T. ) ;
#2870=DIRECTION ( 'NONE',  ( 0.4794255386042042266, 0.000000000000000000, 0.8775825618903720926 ) ) ;
#2880=VERTEX_POINT ( 'NONE', #25156 ) ;
#2887=ORIENTED_EDGE ( 'NONE', *, *, #24848, .F. ) ;
#2907=EDGE_LOOP ( 'NONE', ( #13611, #23142, #26239, #26486 ) ) ;
#2948=DIRECTION ( 'NONE',  ( 1.000000000000000000, 0.000000000000000000, 0.000000000000000000 ) ) ;
#2960=CYLINDRICAL_SURFACE ( 'NONE', #316, 53.34999999999998721 ) ;
#2975=DIRECTION ( 'NONE',  ( 0.8775825618903722036, 0.000000000000000000, -0.4794255386042041156 ) ) ;
#2986=VERTEX_POINT ( 'NONE', #23391 ) ;
#2992=ADVANCED_FACE ( 'NONE', ( #16679 ), #1131, .T. ) ;
#2995=CIRCLE ( 'NONE', #8084, 55.67692378859999991 ) ;
#3001=ORIENTED_EDGE ( 'NONE', *, *, #15191, .T. ) ;
#3015=ORIENTED_EDGE ( 'NONE', *, *, #26696, .T. ) ;
#3016=CONICAL_SURFACE ( 'NONE', #18352, 55.67692378859999280, 1.047197551199999799 ) ;
#3022=ORIENTED_EDGE ( 'NONE', *, *, #4676, .F. ) ;
#3025=DIRECTION ( 'NONE',  ( 0.000000000000000000, 1.000000000000000000, 0.000000000000000000 ) ) ;
#3027=ADVANCED_FACE ( 'NONE', ( #16547 ), #3570, .T. ) ;
#3028=VECTOR ( 'NONE', #9528, 999.9999999999998863 ) ;
#3035=CARTESIAN_POINT ( 'NONE',  ( 0.000000000000000000, -2.000000000000000000, 0.000000000000000000 ) ) ;
#3037=DIRECTION ( 'NONE',  ( 0.000000000000000000, 1.000000000000000000, 0.000000000000000000 ) ) ;
#3053=ORIENTED_EDGE ( 'NONE', *, *, #27993, .T. ) ;
#3055=DIRECTION ( 'NONE',  ( 0.4794255386042037270, 0.000000000000000000, 0.8775825618903724257 ) ) ;
#3058=CONICAL_SURFACE ( 'NONE', #9988, 8.099999999999997868, 0.7853981633970000820 ) ;
#3071=ORIENTED_EDGE ( 'NONE', *, *, #21876, .F. ) ;
#3078=DIRECTION ( 'NONE',  ( 0.000000000000000000, 1.000000000000000000, 0.000000000000000000 ) ) ;
#3083=DIRECTION ( 'NONE',  ( 0.4794255386042040601, 0.000000000000000000, 0.8775825618903720926 ) ) ;
#3106=CARTESIAN_POINT ( 'NONE',  ( 0.000000000000000000, -26.59999999999999787, 0.000000000000000000 ) ) ;
#3119=DIRECTION ( 'NONE',  ( 0.4794255386042036715, 0.000000000000000000, 0.8775825618903724257 ) ) ;
#3137=CARTESIAN_POINT ( 'NONE',  ( -27.18988201479999844, -29.29844555429999886, -49.77074518290000071 ) ) ;
#3140=DIRECTION ( 'NONE',  ( 1.000000000000000000, 0.000000000000000000, 0.000000000000000000 ) ) ;
#3152=DIRECTION ( 'NONE',  ( 0.000000000000000000, 1.000000000000000000, 0.000000000000000000 ) ) ;
#3155=CARTESIAN_POINT ( 'NONE',  ( 0.000000000000000000, -10.00000000000000000, 0.000000000000000000 ) ) ;
#3158=AXIS2_PLACEMENT_3D ( 'NONE', #10884, #19794, #26509 ) ;
#3185=ORIENTED_EDGE ( 'NONE', *, *, #14572, .F. ) ;
#3186=FACE_OUTER_BOUND ( 'NONE', #2506, .T. ) ;
#3187=CARTESIAN_POINT ( 'NONE',  ( -1.598721155459999804E-14, -15.00000000000000000, 50.00000000000000000 ) ) ;
#3189=VERTEX_POINT ( 'NONE', #25154 ) ;
#3195=ORIENTED_EDGE ( 'NONE', *, *, #5913, .T. ) ;
#3199=EDGE_LOOP ( 'NONE', ( #20621, #26057, #23347, #1933 ) ) ;
#3207=FACE_OUTER_BOUND ( 'NONE', #25041, .T. ) ;
#3222=ORIENTED_EDGE ( 'NONE', *, *, #5155, .F. ) ;
#3227=EDGE_LOOP ( 'NONE', ( #7343, #12352, #7592, #21982 ) ) ;
#3244=EDGE_CURVE ( 'NONE', #25772, #28370, #6469, .T. ) ;
#3252=AXIS2_PLACEMENT_3D ( 'NONE', #11099, #28743, #8782 ) ;
#3253=ADVANCED_FACE ( 'NONE', ( #5468 ), #6947, .T. ) ;
#3254=VERTEX_POINT ( 'NONE', #18882 ) ;
#3262=CARTESIAN_POINT ( 'NONE',  ( 25.34421590619999876, -10.95575221240000019, 46.39227603280000523 ) ) ;
#3275=DIRECTION ( 'NONE',  ( 1.000000000000000000, 0.000000000000000000, 0.000000000000000000 ) ) ;
#3276=AXIS2_PLACEMENT_3D ( 'NONE', #6822, #4781, #24889 ) ;
#3278=EDGE_CURVE ( 'NONE', #26635, #12535, #12296, .T. ) ;
#3279=LINE ( 'NONE', #11994, #9665 ) ;
#3289=LINE ( 'NONE', #9959, #1519 ) ;
#3304=DIRECTION ( 'NONE',  ( 0.000000000000000000, 1.000000000000000000, 0.000000000000000000 ) ) ;
#3309=CIRCLE ( 'NONE', #25615, 0.4999999999999990008 ) ;
#3311=AXIS2_PLACEMENT_3D ( 'NONE', #22567, #17751, #6823 ) ;
#3320=CARTESIAN_POINT ( 'NONE',  ( -31.00000000000000000, -11.00000000000000000, -2.486899575159999765E-14 ) ) ;
#3321=EDGE_LOOP ( 'NONE', ( #21756, #13298, #26410, #6339 ) ) ;
#3327=TOROIDAL_SURFACE ( 'NONE', #28419, 55.85192378860000417, 0.3499999999999999778 ) ;
#3336=EDGE_LOOP ( 'NONE', ( #25336, #17133, #10156, #5233 ) ) ;
#3337=CARTESIAN_POINT ( 'NONE',  ( 0.000000000000000000, -19.70310889130000120, 0.000000000000000000 ) ) ;
#3339=DIRECTION ( 'NONE',  ( -0.000000000000000000, 1.000000000000000000, 0.000000000000000000 ) ) ;
#3355=LINE ( 'NONE', #10297, #24912 ) ;
#3362=AXIS2_PLACEMENT_3D ( 'NONE', #18592, #21476, #14759 ) ;
#3365=DIRECTION ( 'NONE',  ( 1.000000000000000000, 0.000000000000000000, 0.000000000000000000 ) ) ;
#3374=EDGE_CURVE ( 'NONE', #16418, #26990, #27885, .T. ) ;
#3386=CARTESIAN_POINT ( 'NONE',  ( -26.77683864449999973, -23.00000000000000000, -49.01467436490000296 ) ) ;
#3391=DIRECTION ( 'NONE',  ( 0.4794255386042036715, 0.000000000000000000, 0.8775825618903724257 ) ) ;
#3392=ORIENTED_EDGE ( 'NONE', *, *, #11965, .F. ) ;
#3406=VECTOR ( 'NONE', #4224, 1000.000000000000000 ) ;
#3413=CARTESIAN_POINT ( 'NONE',  ( 0.000000000000000000, -16.50000000000000000, 0.000000000000000000 ) ) ;
#3429=CARTESIAN_POINT ( 'NONE',  ( 26.69293917519999937, -19.09689110869999951, 48.86109741659999628 ) ) ;
#3432=DIRECTION ( 'NONE',  ( 0.000000000000000000, 1.000000000000000000, 0.000000000000000000 ) ) ;
#3435=ORIENTED_EDGE ( 'NONE', *, *, #26209, .T. ) ;
#3442=CARTESIAN_POINT ( 'NONE',  ( -40.50000000000000000, -15.00000000000000000, 4.500000000000000000 ) ) ;
#3448=VERTEX_POINT ( 'NONE', #2826 ) ;
#3460=ORIENTED_EDGE ( 'NONE', *, *, #26996, .F. ) ;
#3466=EDGE_CURVE ( 'NONE', #3592, #87, #8756, .T. ) ;
#3468=ORIENTED_EDGE ( 'NONE', *, *, #5913, .F. ) ;
#3490=ORIENTED_EDGE ( 'NONE', *, *, #12125, .F. ) ;
#3494=CONICAL_SURFACE ( 'NONE', #8137, 55.67692378859999280, 1.047197551199999799 ) ;
#3501=ORIENTED_EDGE ( 'NONE', *, *, #23788, .T. ) ;
#3506=CARTESIAN_POINT ( 'NONE',  ( 0.000000000000000000, -19.40000000000000213, 0.000000000000000000 ) ) ;
#3513=ORIENTED_EDGE ( 'NONE', *, *, #26160, .T. ) ;
#3526=AXIS2_PLACEMENT_3D ( 'NONE', #13675, #28533, #8568 ) ;
#3532=FACE_OUTER_BOUND ( 'NONE', #8224, .T. ) ;
#3536=VECTOR ( 'NONE', #24102, 999.9999999999998863 ) ;
#3555=ORIENTED_EDGE ( 'NONE', *, *, #17303, .F. ) ;
#3570=CYLINDRICAL_SURFACE ( 'NONE', #28479, 61.34999999999998721 ) ;
#3574=DIRECTION ( 'NONE',  ( 0.000000000000000000, 1.000000000000000000, 0.000000000000000000 ) ) ;
#3592=VERTEX_POINT ( 'NONE', #9474 ) ;
#3605=EDGE_LOOP ( 'NONE', ( #9713, #18793, #7551, #14176 ) ) ;
#3612=EDGE_CURVE ( 'NONE', #13005, #1944, #18520, .T. ) ;
#3618=ORIENTED_EDGE ( 'NONE', *, *, #1656, .F. ) ;
#3627=EDGE_LOOP ( 'NONE', ( #1914, #15490, #4031, #22362 ) ) ;
#3648=DIRECTION ( 'NONE',  ( 0.000000000000000000, -1.000000000000000000, 0.000000000000000000 ) ) ;
#3651=CARTESIAN_POINT ( 'NONE',  ( -27.68682485439999752, -24.80000000000000071, -50.68039294919999804 ) ) ;
#3656=ORIENTED_EDGE ( 'NONE', *, *, #20069, .F. ) ;
#3673=CARTESIAN_POINT ( 'NONE',  ( -25.81706525379999917, -37.08699221940000257, -47.25782095779999992 ) ) ;
#3679=ORIENTED_EDGE ( 'NONE', *, *, #22819, .T. ) ;
#3680=CARTESIAN_POINT ( 'NONE',  ( 0.000000000000000000, -30.50310889129999836, 0.000000000000000000 ) ) ;
#3685=CARTESIAN_POINT ( 'NONE',  ( 0.000000000000000000, -40.00000000000000000, 0.000000000000000000 ) ) ;
#3689=EDGE_CURVE ( 'NONE', #258, #2880, #22282, .T. ) ;
#3700=CARTESIAN_POINT ( 'NONE',  ( -26.77683864449999973, -33.79999999999999716, -49.01467436490000296 ) ) ;
#3707=DIRECTION ( 'NONE',  ( 0.3390050494208429743, 0.7071067811866730279, 0.6205445805637129775 ) ) ;
#3716=DIRECTION ( 'NONE',  ( 0.000000000000000000, 1.000000000000000000, 0.000000000000000000 ) ) ;
#3734=DIRECTION ( 'NONE',  ( 0.000000000000000000, 1.000000000000000000, 0.000000000000000000 ) ) ;
#3735=ORIENTED_EDGE ( 'NONE', *, *, #19657, .F. ) ;
#3742=AXIS2_PLACEMENT_3D ( 'NONE', #25820, #21716, #26380 ) ;
#3745=DIRECTION ( 'NONE',  ( -1.000000000000000000, 0.000000000000000000, -6.123031769109999188E-17 ) ) ;
#3752=VERTEX_POINT ( 'NONE', #20485 ) ;
#3764=CIRCLE ( 'NONE', #24724, 57.75000000000000000 ) ;
#3786=CARTESIAN_POINT ( 'NONE',  ( 0.000000000000000000, -15.50000000000000000, 0.000000000000000000 ) ) ;
#3788=ORIENTED_EDGE ( 'NONE', *, *, #25987, .T. ) ;
#3790=EDGE_CURVE ( 'NONE', #6364, #12325, #4137, .T. ) ;
#3791=CYLINDRICAL_SURFACE ( 'NONE', #20250, 9.500000000000001776 ) ;
#3793=CIRCLE ( 'NONE', #13558, 0.9999999999999980016 ) ;
#3794=CARTESIAN_POINT ( 'NONE',  ( -27.68682485439999752, -24.80000000000000071, -50.68039294919999804 ) ) ;
#3796=FACE_OUTER_BOUND ( 'NONE', #7766, .T. ) ;
#3804=VECTOR ( 'NONE', #8702, 999.9999999999998863 ) ;
#3808=FACE_OUTER_BOUND ( 'NONE', #27249, .T. ) ;
#3813=DIRECTION ( 'NONE',  ( 0.4794255386042041156, 0.000000000000000000, 0.8775825618903720926 ) ) ;
#3841=VERTEX_POINT ( 'NONE', #16331 ) ;
#3844=AXIS2_PLACEMENT_3D ( 'NONE', #17313, #8267, #14423 ) ;
#3849=EDGE_CURVE ( 'NONE', #11391, #17271, #11098, .T. ) ;
#3853=DIRECTION ( 'NONE',  ( 0.000000000000000000, 1.000000000000000000, 0.000000000000000000 ) ) ;
#3871=ORIENTED_EDGE ( 'NONE', *, *, #27031, .F. ) ;
#3878=ADVANCED_FACE ( 'NONE', ( #27712 ), #8262, .T. ) ;
#3886=CARTESIAN_POINT ( 'NONE',  ( 0.000000000000000000, -34.10310889129999623, 0.000000000000000000 ) ) ;
#3892=CIRCLE ( 'NONE', #27660, 9.500000000000001776 ) ;
#3907=ORIENTED_EDGE ( 'NONE', *, *, #6058, .T. ) ;
#3911=EDGE_CURVE ( 'NONE', #640, #13903, #412, .T. ) ;
#3927=DIRECTION ( 'NONE',  ( 0.4794255386042040046, 0.000000000000000000, 0.8775825618903722036 ) ) ;
#3942=EDGE_CURVE ( 'NONE', #4043, #7539, #2730, .T. ) ;
#3981=CARTESIAN_POINT ( 'NONE',  ( 0.000000000000000000, -35.29999999999999716, 0.000000000000000000 ) ) ;
#3994=DIRECTION ( 'NONE',  ( 0.000000000000000000, 1.000000000000000000, 0.000000000000000000 ) ) ;
#4004=EDGE_CURVE ( 'NONE', #20846, #10652, #27375, .T. ) ;
#4010=ADVANCED_FACE ( 'NONE', ( #22134 ), #6384, .T. ) ;
#4012=VERTEX_POINT ( 'NONE', #1610 ) ;
#4024=CARTESIAN_POINT ( 'NONE',  ( 27.68682485439999752, -24.80000000000000071, 50.68039294919999804 ) ) ;
#4031=ORIENTED_EDGE ( 'NONE', *, *, #1746, .T. ) ;
#4043=VERTEX_POINT ( 'NONE', #2033 ) ;
#4066=VECTOR ( 'NONE', #9857, 1000.000000000000000 ) ;
#4071=CARTESIAN_POINT ( 'NONE',  ( -27.18988201479999844, -14.89844555430000028, -49.77074518290000071 ) ) ;
#4079=PRODUCT_DEFINITION_SHAPE ( 'NONE', 'NONE',  #26287 ) ;
#4107=EDGE_CURVE ( 'NONE', #27931, #54, #10133, .T. ) ;
#4129=AXIS2_PLACEMENT_3D ( 'NONE', #13062, #4483, #6676 ) ;
#4137=CIRCLE ( 'NONE', #25110, 24.40223267850000255 ) ;
#4161=DIRECTION ( 'NONE',  ( 0.000000000000000000, 1.000000000000000000, 0.000000000000000000 ) ) ;
#4166=ORIENTED_EDGE ( 'NONE', *, *, #9964, .T. ) ;
#4199=DIRECTION ( 'NONE',  ( 0.4794255386042040601, 0.000000000000000000, 0.8775825618903720926 ) ) ;
#4224=DIRECTION ( 'NONE',  ( 1.000000000000000000, 0.000000000000000000, 0.000000000000000000 ) ) ;
#4226=LINE ( 'NONE', #19525, #8440 ) ;
#4233=AXIS2_PLACEMENT_3D ( 'NONE', #5450, #14333, #3275 ) ;
#4238=CARTESIAN_POINT ( 'NONE',  ( 4.500000000000000000, -11.00000000000000000, -40.50000000000000000 ) ) ;
#4239=AXIS2_PLACEMENT_3D ( 'NONE', #2565, #11414, #20315 ) ;
#4242=FACE_OUTER_BOUND ( 'NONE', #6855, .T. ) ;
#4249=DIRECTION ( 'NONE',  ( 0.4794255386042000078, 0.000000000000000000, 0.8775825618903743131 ) ) ;
#4257=TOROIDAL_SURFACE ( 'NONE', #6596, 60.85000000000000142, 0.5000000000000000000 ) ;
#4258=CIRCLE ( 'NONE', #24270, 0.9999999999999980016 ) ;
#4260=DIRECTION ( 'NONE',  ( 0.4794255386042040046, 0.000000000000000000, 0.8775825618903722036 ) ) ;
#4275=EDGE_CURVE ( 'NONE', #22021, #12657, #9696, .T. ) ;
#4278=DIRECTION ( 'NONE',  ( 0.000000000000000000, 1.000000000000000000, 0.000000000000000000 ) ) ;
#4289=DIRECTION ( 'NONE',  ( 0.4794255386042040046, 0.000000000000000000, 0.8775825618903722036 ) ) ;
#4312=CYLINDRICAL_SURFACE ( 'NONE', #15781, 9.500000000000001776 ) ;
#4321=DIRECTION ( 'NONE',  ( 0.000000000000000000, 1.000000000000000000, 0.000000000000000000 ) ) ;
#4325=ORIENTED_EDGE ( 'NONE', *, *, #10370, .T. ) ;
#4327=CARTESIAN_POINT ( 'NONE',  ( 0.000000000000000000, -23.00000000000000000, 0.000000000000000000 ) ) ;
#4333=CIRCLE ( 'NONE', #8958, 0.4999999999999981126 ) ;
#4337=EDGE_LOOP ( 'NONE', ( #16167, #17740, #7822, #7304 ) ) ;
#4349=DIRECTION ( 'NONE',  ( 1.000000000000000000, 0.000000000000000000, 0.000000000000000000 ) ) ;
#4371=AXIS2_PLACEMENT_3D ( 'NONE', #1114, #5316, #7661 ) ;
#4378=ORIENTED_EDGE ( 'NONE', *, *, #23973, .F. ) ;
#4391=DIRECTION ( 'NONE',  ( 1.000000000000000000, 0.000000000000000000, 0.000000000000000000 ) ) ;
#4393=ORIENTED_EDGE ( 'NONE', *, *, #8059, .F. ) ;
#4394=AXIS2_PLACEMENT_3D ( 'NONE', #22250, #13346, #16122 ) ;
#4400=AXIS2_PLACEMENT_3D ( 'NONE', #4895, #17865, #24418 ) ;
#4406=DIRECTION ( 'NONE',  ( 0.4794255386042000078, 0.000000000000000000, 0.8775825618903743131 ) ) ;
#4411=AXIS2_PLACEMENT_3D ( 'NONE', #5838, #14721, #174 ) ;
#4413=ORIENTED_EDGE ( 'NONE', *, *, #5538, .F. ) ;
#4416=CARTESIAN_POINT ( 'NONE',  ( 4.362772401299999991, -17.50000000000000000, 7.986001313199998286 ) ) ;
#4417=ORIENTED_EDGE ( 'NONE', *, *, #20782, .T. ) ;
#4429=DIRECTION ( 'NONE',  ( -0.8775825618903722036, 0.000000000000000000, 0.4794255386042041156 ) ) ;
#4430=DIRECTION ( 'NONE',  ( 0.4794255386042040601, 0.000000000000000000, 0.8775825618903720926 ) ) ;
#4444=FACE_OUTER_BOUND ( 'NONE', #8413, .T. ) ;
#4448=CIRCLE ( 'NONE', #20765, 60.85000000000000142 ) ;
#4454=DIRECTION ( 'NONE',  ( 1.000000000000000000, 0.000000000000000000, 0.000000000000000000 ) ) ;
#4456=DIRECTION ( 'NONE',  ( 0.000000000000000000, 1.000000000000000000, 0.000000000000000000 ) ) ;
#4458=AXIS2_PLACEMENT_3D ( 'NONE', #20579, #20876, #5280 ) ;
#4459=CARTESIAN_POINT ( 'NONE',  ( 0.000000000000000000, -11.00000000000000000, 24.50000000000000000 ) ) ;
#4480=ORIENTED_EDGE ( 'NONE', *, *, #22135, .T. ) ;
#4483=DIRECTION ( 'NONE',  ( 0.000000000000000000, 1.000000000000000000, 0.000000000000000000 ) ) ;
#4545=CONICAL_SURFACE ( 'NONE', #398, 24.40223267850002031, 0.7949521073230001456 ) ;
#4553=CONICAL_SURFACE ( 'NONE', #24565, 55.67692378859999280, 1.047197551199999799 ) ;
#4569=LINE ( 'NONE', #8929, #11088 ) ;
#4586=ORIENTED_EDGE ( 'NONE', *, *, #11404, .T. ) ;
#4591=CARTESIAN_POINT ( 'NONE',  ( -27.18988201479999844, -34.70155444569999759, -49.77074518290000071 ) ) ;
#4599=DIRECTION ( 'NONE',  ( 3.652049423109066841E-16, 0.000000000000000000, -1.000000000000000000 ) ) ;
#4628=VERTEX_POINT ( 'NONE', #24594 ) ;
#4629=ORIENTED_EDGE ( 'NONE', *, *, #5318, .F. ) ;
#4637=DIRECTION ( 'NONE',  ( 0.000000000000000000, 1.000000000000000000, 0.000000000000000000 ) ) ;
#4639=CIRCLE ( 'NONE', #23709, 0.3500000000000003664 ) ;
#4644=CARTESIAN_POINT ( 'NONE',  ( 26.77683864449999973, -26.59999999999999787, 49.01467436490000296 ) ) ;
#4646=CARTESIAN_POINT ( 'NONE',  ( 0.000000000000000000, -16.00000000000000000, 0.000000000000000000 ) ) ;
#4651=CARTESIAN_POINT ( 'NONE',  ( 0.000000000000000000, -36.20000000000000284, 0.000000000000000000 ) ) ;
#4655=CARTESIAN_POINT ( 'NONE',  ( 0.000000000000000000, -13.40000000000000036, 0.000000000000000000 ) ) ;
#4659=AXIS2_PLACEMENT_3D ( 'NONE', #28136, #18697, #3391 ) ;
#4665=LINE ( 'NONE', #8718, #7501 ) ;
#4672=CARTESIAN_POINT ( 'NONE',  ( 4.500000000000000000, -15.00000000000000000, -50.00000000000000000 ) ) ;
#4674=VERTEX_POINT ( 'NONE', #28653 ) ;
#4676=EDGE_CURVE ( 'NONE', #11154, #2880, #26949, .T. ) ;
#4680=AXIS2_PLACEMENT_3D ( 'NONE', #2723, #18153, #11577 ) ;
#4681=DIRECTION ( 'NONE',  ( 0.4794255386042040601, 0.000000000000000000, 0.8775825618903720926 ) ) ;
#4700=AXIS2_PLACEMENT_3D ( 'NONE', #3673, #10484, #8050 ) ;
#4708=CARTESIAN_POINT ( 'NONE',  ( 0.000000000000000000, -40.00000000000000000, 0.000000000000000000 ) ) ;
#4711=EDGE_CURVE ( 'NONE', #20961, #14272, #2295, .T. ) ;
#4714=DIRECTION ( 'NONE',  ( 0.000000000000000000, 1.000000000000000000, 0.000000000000000000 ) ) ;
#4732=AXIS2_PLACEMENT_3D ( 'NONE', #171, #17926, #26817 ) ;
#4744=AXIS2_PLACEMENT_3D ( 'NONE', #17099, #23661, #12991 ) ;
#4750=AXIS2_PLACEMENT_3D ( 'NONE', #1174, #3339, #14405 ) ;
#4757=DIRECTION ( 'NONE',  ( 1.000000000000000000, 0.000000000000000000, 0.000000000000000000 ) ) ;
#4765=CARTESIAN_POINT ( 'NONE',  ( 0.000000000000000000, -33.79999999999999716, 0.000000000000000000 ) ) ;
#4773=EDGE_LOOP ( 'NONE', ( #28293, #9989 ) ) ;
#4774=AXIS2_PLACEMENT_3D ( 'NONE', #7797, #18586, #16385 ) ;
#4781=DIRECTION ( 'NONE',  ( 0.000000000000000000, 1.000000000000000000, 0.000000000000000000 ) ) ;
#4790=DIRECTION ( 'NONE',  ( 0.000000000000000000, 1.000000000000000000, 0.000000000000000000 ) ) ;
#4801=CARTESIAN_POINT ( 'NONE',  ( 31.00000000000000000, -15.00000000000000000, 4.500000000000000000 ) ) ;
#4804=AXIS2_PLACEMENT_3D ( 'NONE', #16954, #25845, #5867 ) ;
#4808=CARTESIAN_POINT ( 'NONE',  ( 0.000000000000000000, -19.40000000000000213, 0.000000000000000000 ) ) ;
#4817=ADVANCED_FACE ( 'NONE', ( #16572 ), #12187, .F. ) ;
#4820=ORIENTED_EDGE ( 'NONE', *, *, #16351, .T. ) ;
#4837=FACE_OUTER_BOUND ( 'NONE', #3336, .T. ) ;
#4840=ORIENTED_EDGE ( 'NONE', *, *, #19218, .T. ) ;
#4874=DIRECTION ( 'NONE',  ( 1.000000000000000000, 0.000000000000000000, 0.000000000000000000 ) ) ;
#4895=CARTESIAN_POINT ( 'NONE',  ( 0.000000000000000000, -15.50000000000000000, 0.000000000000000000 ) ) ;
#4896=DIRECTION ( 'NONE',  ( 0.4794255386042059475, 0.000000000000000000, 0.8775825618903710934 ) ) ;
#4900=DIRECTION ( 'NONE',  ( 1.000000000000000000, 0.000000000000000000, 0.000000000000000000 ) ) ;
#4910=ORIENTED_EDGE ( 'NONE', *, *, #27863, .F. ) ;
#4923=DIRECTION ( 'NONE',  ( 1.000000000000000000, 0.000000000000000000, 0.000000000000000000 ) ) ;
#4926=LINE ( 'NONE', #27369, #23411 ) ;
#4928=DIRECTION ( 'NONE',  ( 0.4794255386042036715, 0.000000000000000000, 0.8775825618903722036 ) ) ;
#4931=ORIENTED_EDGE ( 'NONE', *, *, #23143, .T. ) ;
#4945=DIRECTION ( 'NONE',  ( 0.4794255386042036715, 0.000000000000000000, 0.8775825618903724257 ) ) ;
#4950=AXIS2_PLACEMENT_3D ( 'NONE', #19829, #17808, #22178 ) ;
#4972=ORIENTED_EDGE ( 'NONE', *, *, #10120, .T. ) ;
#4977=EDGE_CURVE ( 'NONE', #18448, #14011, #4569, .T. ) ;
#4987=DIRECTION ( 'NONE',  ( 0.000000000000000000, 1.000000000000000000, 0.000000000000000000 ) ) ;
#4998=VERTEX_POINT ( 'NONE', #17545 ) ;
#5005=FACE_OUTER_BOUND ( 'NONE', #27732, .T. ) ;
#5013=EDGE_CURVE ( 'NONE', #15673, #6736, #11568, .T. ) ;
#5021=CIRCLE ( 'NONE', #14344, 0.3500000000000003664 ) ;
#5040=AXIS2_PLACEMENT_3D ( 'NONE', #3886, #14804, #1711 ) ;
#5044=ORIENTED_EDGE ( 'NONE', *, *, #9159, .T. ) ;
#5046=DIRECTION ( 'NONE',  ( 0.000000000000000000, 1.000000000000000000, 0.000000000000000000 ) ) ;
#5050=DIRECTION ( 'NONE',  ( 0.000000000000000000, 1.000000000000000000, 0.000000000000000000 ) ) ;
#5066=DIRECTION ( 'NONE',  ( 0.4794255386042000078, 0.000000000000000000, 0.8775825618903743131 ) ) ;
#5068=EDGE_CURVE ( 'NONE', #5395, #15179, #25417, .T. ) ;
#5071=FACE_OUTER_BOUND ( 'NONE', #27797, .T. ) ;
#5073=ADVANCED_FACE ( 'NONE', ( #9523 ), #16239, .T. ) ;
#5075=VERTEX_POINT ( 'NONE', #526 ) ;
#5085=EDGE_LOOP ( 'NONE', ( #10608, #16930 ) ) ;
#5094=CARTESIAN_POINT ( 'NONE',  ( 4.500000000000000000, -15.00000000000000000, 31.00000000000000000 ) ) ;
#5102=ORIENTED_EDGE ( 'NONE', *, *, #12897, .T. ) ;
#5105=AXIS2_PLACEMENT_3D ( 'NONE', #7315, #7475, #20869 ) ;
#5109=VERTEX_POINT ( 'NONE', #16521 ) ;
#5111=CARTESIAN_POINT ( 'NONE',  ( -50.00000000000000000, -12.50000000000000000, 4.500000000000000000 ) ) ;
#5112=CIRCLE ( 'NONE', #26037, 57.75000000000000000 ) ;
#5114=AXIS2_PLACEMENT_3D ( 'NONE', #27613, #14197, #7781 ) ;
#5118=EDGE_CURVE ( 'NONE', #11046, #6607, #12538, .T. ) ;
#5123=LINE ( 'NONE', #25240, #20931 ) ;
#5127=ORIENTED_EDGE ( 'NONE', *, *, #16186, .F. ) ;
#5128=DIRECTION ( 'NONE',  ( 1.000000000000000000, 0.000000000000000000, 0.000000000000000000 ) ) ;
#5131=ORIENTED_EDGE ( 'NONE', *, *, #8271, .T. ) ;
#5153=ORIENTED_EDGE ( 'NONE', *, *, #19348, .F. ) ;
#5154=CONICAL_SURFACE ( 'NONE', #8839, 55.67692378859999280, 1.047197551199999799 ) ;
#5155=EDGE_CURVE ( 'NONE', #21247, #16409, #19401, .T. ) ;
#5162=DIRECTION ( 'NONE',  ( -0.4151946956541399669, 0.5000000000001689759, -0.7600087925152558821 ) ) ;
#5173=CIRCLE ( 'NONE', #11664, 0.3500000000000003664 ) ;
#5184=DIRECTION ( 'NONE',  ( 0.000000000000000000, 1.000000000000000000, 0.000000000000000000 ) ) ;
#5186=ORIENTED_EDGE ( 'NONE', *, *, #11965, .T. ) ;
#5195=CIRCLE ( 'NONE', #984, 0.4999999999999981126 ) ;
#5200=CYLINDRICAL_SURFACE ( 'NONE', #6943, 57.74999999999999289 ) ;
#5208=DIRECTION ( 'NONE',  ( 0.000000000000000000, 1.000000000000000000, 0.000000000000000000 ) ) ;
#5211=DIRECTION ( 'NONE',  ( -0.4381045938801422235, -0.4061384660531317525, -0.8019450799232605842 ) ) ;
#5216=ADVANCED_FACE ( 'NONE', ( #13412 ), #23249, .F. ) ;
#5219=CARTESIAN_POINT ( 'NONE',  ( 0.000000000000000000, -17.30000000000000071, 0.000000000000000000 ) ) ;
#5229=DIRECTION ( 'NONE',  ( 0.000000000000000000, 1.000000000000000000, 0.000000000000000000 ) ) ;
#5233=ORIENTED_EDGE ( 'NONE', *, *, #7346, .F. ) ;
#5245=CARTESIAN_POINT ( 'NONE',  ( 29.41275679339999982, -10.50000000000000000, 53.83969017199999740 ) ) ;
#5255=AXIS2_PLACEMENT_3D ( 'NONE', #25032, #5366, #5066 ) ;
#5264=DIRECTION ( 'NONE',  ( 1.000000000000000000, 0.000000000000000000, 0.000000000000000000 ) ) ;
#5270=DIRECTION ( 'NONE',  ( 0.4794255386042036715, 0.000000000000000000, 0.8775825618903724257 ) ) ;
#5278=TOROIDAL_SURFACE ( 'NONE', #2002, 55.85192378860000417, 0.3499999999999999778 ) ;
#5280=DIRECTION ( 'NONE',  ( 0.4794255386042000078, 0.000000000000000000, 0.8775825618903743131 ) ) ;
#5286=EDGE_CURVE ( 'NONE', #16026, #20739, #8794, .T. ) ;
#5315=LINE ( 'NONE', #14205, #3028 ) ;
#5316=DIRECTION ( 'NONE',  ( 0.000000000000000000, 1.000000000000000000, 0.000000000000000000 ) ) ;
#5318=EDGE_CURVE ( 'NONE', #77, #7539, #13941, .T. ) ;
#5324=EDGE_CURVE ( 'NONE', #19945, #25155, #14402, .T. ) ;
#5331=LINE ( 'NONE', #20636, #14500 ) ;
#5336=VERTEX_POINT ( 'NONE', #7176 ) ;
#5344=VECTOR ( 'NONE', #23415, 1000.000000000000000 ) ;
#5346=ADVANCED_FACE ( 'NONE', ( #27135 ), #21826, .F. ) ;
#5351=ADVANCED_FACE ( 'NONE', ( #22915 ), #25127, .T. ) ;
#5354=AXIS2_PLACEMENT_3D ( 'NONE', #2241, #370, #7058 ) ;
#5365=ORIENTED_EDGE ( 'NONE', *, *, #11712, .T. ) ;
#5366=DIRECTION ( 'NONE',  ( -0.8775825618903722036, 0.000000000000000000, 0.4794255386042041156 ) ) ;
#5370=CIRCLE ( 'NONE', #16046, 61.35000000000000142 ) ;
#5385=EDGE_CURVE ( 'NONE', #20961, #23467, #14675, .T. ) ;
#5395=VERTEX_POINT ( 'NONE', #25093 ) ;
#5401=CARTESIAN_POINT ( 'NONE',  ( 26.77683864449999973, -15.80000000000000071, 49.01467436490000296 ) ) ;
#5405=LINE ( 'NONE', #18521, #5780 ) ;
#5411=DIRECTION ( 'NONE',  ( 0.000000000000000000, 1.000000000000000000, 0.000000000000000000 ) ) ;
#5420=CARTESIAN_POINT ( 'NONE',  ( 27.68682485439999752, -24.80000000000000071, 50.68039294919999804 ) ) ;
#5444=EDGE_LOOP ( 'NONE', ( #7006, #3460, #15268, #10356 ) ) ;
#5450=CARTESIAN_POINT ( 'NONE',  ( 0.000000000000000000, -13.50000000000000000, 0.000000000000000000 ) ) ;
#5468=FACE_OUTER_BOUND ( 'NONE', #6110, .T. ) ;
#5469=EDGE_LOOP ( 'NONE', ( #3618, #13500, #604, #21670 ) ) ;
#5477=AXIS2_PLACEMENT_3D ( 'NONE', #23785, #12688, #10631 ) ;
#5481=ADVANCED_FACE ( 'NONE', ( #14505 ), #26970, .T. ) ;
#5485=CARTESIAN_POINT ( 'NONE',  ( 0.000000000000000000, -23.00000000000000000, 0.000000000000000000 ) ) ;
#5486=DIRECTION ( 'NONE',  ( 1.000000000000000000, 0.000000000000000000, 0.000000000000000000 ) ) ;
#5503=AXIS2_PLACEMENT_3D ( 'NONE', #12322, #5771, #16568 ) ;
#5529=LINE ( 'NONE', #1456, #18870 ) ;
#5535=DIRECTION ( 'NONE',  ( 0.8775825618903722036, 0.000000000000000000, -0.4794255386042041156 ) ) ;
#5538=EDGE_CURVE ( 'NONE', #9851, #5109, #2137, .T. ) ;
#5540=CARTESIAN_POINT ( 'NONE',  ( 0.000000000000000000, -34.10310889129999623, 0.000000000000000000 ) ) ;
#5543=CARTESIAN_POINT ( 'NONE',  ( -10.35605037799999906, -12.64149019679999952, -18.95662306240000206 ) ) ;
#5545=CIRCLE ( 'NONE', #12498, 9.099999999999999645 ) ;
#5557=DIRECTION ( 'NONE',  ( 0.000000000000000000, 1.000000000000000000, 0.000000000000000000 ) ) ;
#5560=DIRECTION ( 'NONE',  ( 0.000000000000000000, -1.000000000000000000, 0.000000000000000000 ) ) ;
#5562=DIRECTION ( 'NONE',  ( 0.000000000000000000, 0.000000000000000000, 1.000000000000000000 ) ) ;
#5564=AXIS2_PLACEMENT_3D ( 'NONE', #28647, #13348, #24438 ) ;
#5566=AXIS2_PLACEMENT_3D ( 'NONE', #6868, #10909, #19964 ) ;
#5573=EDGE_CURVE ( 'NONE', #28180, #5596, #8178, .T. ) ;
#5577=DIRECTION ( 'NONE',  ( 0.000000000000000000, 1.000000000000000000, 0.000000000000000000 ) ) ;
#5587=DIRECTION ( 'NONE',  ( -1.836909530729999990E-16, 0.000000000000000000, 1.000000000000000000 ) ) ;
#5589=AXIS2_PLACEMENT_3D ( 'NONE', #24592, #20361, #432 ) ;
#5596=VERTEX_POINT ( 'NONE', #9984 ) ;
#5612=DIRECTION ( 'NONE',  ( 0.000000000000000000, 1.000000000000000000, 0.000000000000000000 ) ) ;
#5614=DIRECTION ( 'NONE',  ( 1.000000000000000000, 0.000000000000000000, 0.000000000000000000 ) ) ;
#5617=CARTESIAN_POINT ( 'NONE',  ( 0.000000000000000000, -22.69689110870000093, 0.000000000000000000 ) ) ;
#5626=DIRECTION ( 'NONE',  ( 0.4151946956541399669, 0.5000000000001689759, 0.7600087925152558821 ) ) ;
#5630=EDGE_CURVE ( 'NONE', #24400, #20739, #25871, .T. ) ;
#5635=EDGE_CURVE ( 'NONE', #1856, #14426, #5847, .T. ) ;
#5650=LINE ( 'NONE', #17140, #12716 ) ;
#5677=DIRECTION ( 'NONE',  ( 0.000000000000000000, 1.000000000000000000, 0.000000000000000000 ) ) ;
#5679=CONICAL_SURFACE ( 'NONE', #7583, 55.67692378859999280, 1.047197551199999799 ) ;
#5688=CARTESIAN_POINT ( 'NONE',  ( 0.000000000000000000, -15.80000000000000071, 0.000000000000000000 ) ) ;
#5694=DIRECTION ( 'NONE',  ( -0.8775825618903722036, 0.000000000000000000, 0.4794255386042041156 ) ) ;
#5701=ORIENTED_EDGE ( 'NONE', *, *, #10987, .T. ) ;
#5733=EDGE_CURVE ( 'NONE', #8975, #15620, #16574, .T. ) ;
#5736=LINE ( 'NONE', #14620, #27138 ) ;
#5754=VECTOR ( 'NONE', #3853, 1000.000000000000000 ) ;
#5762=CIRCLE ( 'NONE', #16460, 55.67692378859999991 ) ;
#5771=DIRECTION ( 'NONE',  ( 0.000000000000000000, 1.000000000000000000, 0.000000000000000000 ) ) ;
#5780=VECTOR ( 'NONE', #13998, 999.9999999999998863 ) ;
#5782=ORIENTED_EDGE ( 'NONE', *, *, #3942, .F. ) ;
#5808=ORIENTED_EDGE ( 'NONE', *, *, #4004, .T. ) ;
#5816=CARTESIAN_POINT ( 'NONE',  ( 50.00000000000000000, -11.00000000000000000, 1.776356839399999922E-14 ) ) ;
#5830=EDGE_CURVE ( 'NONE', #10454, #16409, #15138, .T. ) ;
#5833=CARTESIAN_POINT ( 'NONE',  ( 29.08514934200000113, -20.00000000000000000, 53.24000875469999983 ) ) ;
#5838=CARTESIAN_POINT ( 'NONE',  ( 6.831813925109999630, -11.50000000000000000, 12.50555150689999984 ) ) ;
#5847=CIRCLE ( 'NONE', #10041, 53.75557630320000868 ) ;
#5867=DIRECTION ( 'NONE',  ( 0.000000000000000000, 0.000000000000000000, 1.000000000000000000 ) ) ;
#5883=CARTESIAN_POINT ( 'NONE',  ( 0.000000000000000000, -20.00000000000000000, 0.000000000000000000 ) ) ;
#5904=DIRECTION ( 'NONE',  ( 1.000000000000000000, 0.000000000000000000, 0.000000000000000000 ) ) ;
#5906=CARTESIAN_POINT ( 'NONE',  ( 40.50000000000000000, -15.00000000000000000, -4.500000000000000000 ) ) ;
#5910=ORIENTED_EDGE ( 'NONE', *, *, #14064, .F. ) ;
#5912=SHAPE_REPRESENTATION ( 'Serpentine Belt Drive Pulley', ( #26433 ), #1786 ) ;
#5913=EDGE_CURVE ( 'NONE', #18617, #22563, #16626, .T. ) ;
#5930=ADVANCED_FACE ( 'NONE', ( #16343 ), #7756, .T. ) ;
#5933=EDGE_CURVE ( 'NONE', #18741, #19945, #25873, .T. ) ;
#5942=EDGE_LOOP ( 'NONE', ( #6451, #8534, #17650, #11971 ) ) ;
#5959=CARTESIAN_POINT ( 'NONE',  ( 0.000000000000000000, -15.49689110870000164, 0.000000000000000000 ) ) ;
#5960=FACE_OUTER_BOUND ( 'NONE', #23476, .T. ) ;
#5961=DIRECTION ( 'NONE',  ( 0.000000000000000000, 1.000000000000000000, 0.000000000000000000 ) ) ;
#5965=EDGE_CURVE ( 'NONE', #7778, #2153, #786, .T. ) ;
#5980=VECTOR ( 'NONE', #25647, 1000.000000000000000 ) ;
#5981=CYLINDRICAL_SURFACE ( 'NONE', #21598, 57.74999999999999289 ) ;
#5984=ORIENTED_EDGE ( 'NONE', *, *, #26451, .T. ) ;
#5988=EDGE_LOOP ( 'NONE', ( #1957, #26836, #6921, #13735 ) ) ;
#5994=DIRECTION ( 'NONE',  ( 0.8775825618903722036, 0.000000000000000000, -0.4794255386042041156 ) ) ;
#6013=ADVANCED_FACE ( 'NONE', ( #18690 ), #2960, .F. ) ;
#6014=DIRECTION ( 'NONE',  ( 0.000000000000000000, 1.000000000000000000, 0.000000000000000000 ) ) ;
#6026=DIRECTION ( 'NONE',  ( -0.8775825618903722036, 0.000000000000000000, 0.4794255386042041156 ) ) ;
#6034=TOROIDAL_SURFACE ( 'NONE', #27480, 55.85192378860000417, 0.3499999999999999778 ) ;
#6042=EDGE_CURVE ( 'NONE', #54, #24400, #20309, .T. ) ;
#6047=EDGE_LOOP ( 'NONE', ( #16082, #11663, #8791, #23195 ) ) ;
#6054=TOROIDAL_SURFACE ( 'NONE', #22844, 55.85192378860000417, 0.3499999999999999778 ) ;
#6058=EDGE_CURVE ( 'NONE', #18617, #11029, #6105, .T. ) ;
#6068=EDGE_LOOP ( 'NONE', ( #28569, #17466, #8081, #2714 ) ) ;
#6072=AXIS2_PLACEMENT_3D ( 'NONE', #13634, #16251, #18607 ) ;
#6074=CIRCLE ( 'NONE', #21445, 57.75000000000000000 ) ;
#6079=EDGE_LOOP ( 'NONE', ( #26468, #24749, #5044, #21907 ) ) ;
#6093=DIRECTION ( 'NONE',  ( 1.000000000000000000, 0.000000000000000000, 0.000000000000000000 ) ) ;
#6103=CIRCLE ( 'NONE', #20071, 9.500000000000001776 ) ;
#6105=LINE ( 'NONE', #12650, #803 ) ;
#6107=ADVANCED_FACE ( 'NONE', ( #27844 ), #16168, .F. ) ;
#6110=EDGE_LOOP ( 'NONE', ( #27556, #1357, #19911, #9408 ) ) ;
#6111=VECTOR ( 'NONE', #1286, 1000.000000000000000 ) ;
#6116=CARTESIAN_POINT ( 'NONE',  ( 0.000000000000000000, -32.30000000000000426, 0.000000000000000000 ) ) ;
#6126=EDGE_LOOP ( 'NONE', ( #28719, #6610, #7619, #27446 ) ) ;
#6127=CARTESIAN_POINT ( 'NONE',  ( 0.000000000000000000, -40.00000000000000000, 0.000000000000000000 ) ) ;
#6130=PLANE ( 'NONE',  #24719 ) ;
#6155=EDGE_LOOP ( 'NONE', ( #4378, #10226, #2498, #28763 ) ) ;
#6158=DIRECTION ( 'NONE',  ( 0.000000000000000000, 1.000000000000000000, 0.000000000000000000 ) ) ;
#6170=CARTESIAN_POINT ( 'NONE',  ( 0.000000000000000000, -33.79999999999999716, 0.000000000000000000 ) ) ;
#6174=EDGE_CURVE ( 'NONE', #5109, #9851, #1299, .T. ) ;
#6177=AXIS2_PLACEMENT_3D ( 'NONE', #11377, #7323, #9634 ) ;
#6182=CARTESIAN_POINT ( 'NONE',  ( 0.000000000000000000, -35.29999999999999716, 0.000000000000000000 ) ) ;
#6183=EDGE_LOOP ( 'NONE', ( #9626, #9764, #17749, #6573 ) ) ;
#6184=EDGE_CURVE ( 'NONE', #24319, #3448, #10099, .T. ) ;
#6186=VECTOR ( 'NONE', #23423, 1000.000000000000114 ) ;
#6192=CARTESIAN_POINT ( 'NONE',  ( 0.000000000000000000, -2.000000000000000000, 0.000000000000000000 ) ) ;
#6203=CARTESIAN_POINT ( 'NONE',  ( -50.00000000000000000, -13.00000000000000000, -4.500000000000000000 ) ) ;
#6204=EDGE_CURVE ( 'NONE', #7778, #23820, #24530, .T. ) ;
#6217=ORIENTED_EDGE ( 'NONE', *, *, #6361, .T. ) ;
#6219=AXIS2_PLACEMENT_3D ( 'NONE', #20247, #15862, #13529 ) ;
#6236=VECTOR ( 'NONE', #2431, 1000.000000000000114 ) ;
#6241=EDGE_CURVE ( 'NONE', #17271, #11391, #28236, .T. ) ;
#6243=EDGE_CURVE ( 'NONE', #25155, #19419, #21291, .T. ) ;
#6246=CARTESIAN_POINT ( 'NONE',  ( -4.362772401299999991, -17.50000000000000000, -7.986001313199998286 ) ) ;
#6250=DIRECTION ( 'NONE',  ( 0.4794255386042041156, 0.000000000000000000, 0.8775825618903722036 ) ) ;
#6252=DIRECTION ( 'NONE',  ( 0.000000000000000000, 1.000000000000000000, 0.000000000000000000 ) ) ;
#6260=FACE_OUTER_BOUND ( 'NONE', #28547, .T. ) ;
#6280=CARTESIAN_POINT ( 'NONE',  ( 0.000000000000000000, -11.00000000000000000, 0.000000000000000000 ) ) ;
#6295=ORIENTED_EDGE ( 'NONE', *, *, #4977, .F. ) ;
#6308=DIRECTION ( 'NONE',  ( 0.4794255386042059475, 0.000000000000000000, 0.8775825618903710934 ) ) ;
#6311=EDGE_CURVE ( 'NONE', #584, #8975, #11930, .T. ) ;
#6331=CARTESIAN_POINT ( 'NONE',  ( 0.000000000000000000, -30.20000000000000284, 0.000000000000000000 ) ) ;
#6339=ORIENTED_EDGE ( 'NONE', *, *, #6042, .T. ) ;
#6344=FACE_OUTER_BOUND ( 'NONE', #17753, .T. ) ;
#6353=LINE ( 'NONE', #4024, #9711 ) ;
#6360=ORIENTED_EDGE ( 'NONE', *, *, #7841, .T. ) ;
#6361=EDGE_CURVE ( 'NONE', #26131, #19846, #26042, .T. ) ;
#6364=VERTEX_POINT ( 'NONE', #28089 ) ;
#6373=TOROIDAL_SURFACE ( 'NONE', #6877, 57.54999999999999716, 1.000000000000000000 ) ;
#6384=CYLINDRICAL_SURFACE ( 'NONE', #19009, 57.74999999999999289 ) ;
#6385=CYLINDRICAL_SURFACE ( 'NONE', #11406, 9.500000000000001776 ) ;
#6389=ORIENTED_EDGE ( 'NONE', *, *, #12891, .T. ) ;
#6410=VECTOR ( 'NONE', #5211, 1000.000000000000114 ) ;
#6451=ORIENTED_EDGE ( 'NONE', *, *, #5635, .F. ) ;
#6459=DIRECTION ( 'NONE',  ( 0.000000000000000000, 1.000000000000000000, 0.000000000000000000 ) ) ;
#6465=CONICAL_SURFACE ( 'NONE', #3252, 55.67692378859999280, 1.047197551199999799 ) ;
#6469=CIRCLE ( 'NONE', #26482, 60.66666666670000296 ) ;
#6480=ORIENTED_EDGE ( 'NONE', *, *, #9377, .T. ) ;
#6488=AXIS2_PLACEMENT_3D ( 'NONE', #1033, #5229, #20526 ) ;
#6494=CARTESIAN_POINT ( 'NONE',  ( 27.68682485439999752, -32.30000000000000426, 50.68039294919999804 ) ) ;
#6496=DIRECTION ( 'NONE',  ( 0.000000000000000000, 1.000000000000000000, 0.000000000000000000 ) ) ;
#6503=EDGE_LOOP ( 'NONE', ( #1057, #28231, #20214, #23176 ) ) ;
#6518=EDGE_CURVE ( 'NONE', #20862, #13903, #5736, .T. ) ;
#6529=AXIS2_PLACEMENT_3D ( 'NONE', #27339, #3025, #25159 ) ;
#6532=CIRCLE ( 'NONE', #17704, 6.999999999999999112 ) ;
#6533=AXIS2_PLACEMENT_3D ( 'NONE', #22109, #17297, #26475 ) ;
#6541=FACE_OUTER_BOUND ( 'NONE', #13499, .T. ) ;
#6553=AXIS2_PLACEMENT_3D ( 'NONE', #3386, #18967, #7894 ) ;
#6557=DIRECTION ( 'NONE',  ( 0.000000000000000000, 1.000000000000000000, 0.000000000000000000 ) ) ;
#6558=DIRECTION ( 'NONE',  ( 0.4794255386042041156, 0.000000000000000000, 0.8775825618903720926 ) ) ;
#6565=FACE_OUTER_BOUND ( 'NONE', #17245, .T. ) ;
#6571=VECTOR ( 'NONE', #9807, 1000.000000000000000 ) ;
#6573=ORIENTED_EDGE ( 'NONE', *, *, #9195, .T. ) ;
#6584=ORIENTED_EDGE ( 'NONE', *, *, #1875, .F. ) ;
#6596=AXIS2_PLACEMENT_3D ( 'NONE', #2520, #9633, #11376 ) ;
#6607=VERTEX_POINT ( 'NONE', #546 ) ;
#6610=ORIENTED_EDGE ( 'NONE', *, *, #9903, .F. ) ;
#6631=FACE_OUTER_BOUND ( 'NONE', #14070, .T. ) ;
#6642=DIRECTION ( 'NONE',  ( 0.000000000000000000, 1.000000000000000000, 0.000000000000000000 ) ) ;
#6646=FACE_OUTER_BOUND ( 'NONE', #10732, .T. ) ;
#6649=DIRECTION ( 'NONE',  ( 0.000000000000000000, 1.000000000000000000, 0.000000000000000000 ) ) ;
#6655=CIRCLE ( 'NONE', #143, 53.35000000000000142 ) ;
#6658=VECTOR ( 'NONE', #20963, 1000.000000000000000 ) ;
#6664=VERTEX_POINT ( 'NONE', #3429 ) ;
#6670=ORIENTED_EDGE ( 'NONE', *, *, #6892, .F. ) ;
#6676=DIRECTION ( 'NONE',  ( 1.000000000000000000, 0.000000000000000000, 0.000000000000000000 ) ) ;
#6678=VECTOR ( 'NONE', #22314, 1000.000000000000000 ) ;
#6680=LINE ( 'NONE', #26493, #28522 ) ;
#6684=MANIFOLD_SOLID_BREP ( 'Rotational Bodies', #21651 ) ;
#6686=CARTESIAN_POINT ( 'NONE',  ( 0.000000000000000000, -19.40000000000000213, 0.000000000000000000 ) ) ;
#6712=AXIS2_PLACEMENT_3D ( 'NONE', #14800, #3745, #8382 ) ;
#6725=ORIENTED_EDGE ( 'NONE', *, *, #15743, .T. ) ;
#6736=VERTEX_POINT ( 'NONE', #11871 ) ;
#6738=AXIS2_PLACEMENT_3D ( 'NONE', #10382, #8496, #15175 ) ;
#6748=EDGE_CURVE ( 'NONE', #26131, #25637, #21997, .T. ) ;
#6754=ADVANCED_FACE ( 'NONE', ( #20783 ), #7937, .T. ) ;
#6786=EDGE_CURVE ( 'NONE', #25949, #14280, #11229, .T. ) ;
#6795=CARTESIAN_POINT ( 'NONE',  ( 0.000000000000000000, -2.000000000000000000, 0.000000000000000000 ) ) ;
#6797=FACE_OUTER_BOUND ( 'NONE', #13504, .T. ) ;
#6800=FACE_BOUND ( 'NONE', #16098, .T. ) ;
#6812=CARTESIAN_POINT ( 'NONE',  ( -11.74592569580000045, -14.00000000000000000, -21.50077276629999901 ) ) ;
#6814=DIRECTION ( 'NONE',  ( 0.4794255386042041711, 0.000000000000000000, 0.8775825618903720926 ) ) ;
#6820=CARTESIAN_POINT ( 'NONE',  ( 0.000000000000000000, -40.00000000000000000, 0.000000000000000000 ) ) ;
#6821=ORIENTED_EDGE ( 'NONE', *, *, #4676, .T. ) ;
#6822=CARTESIAN_POINT ( 'NONE',  ( 0.000000000000000000, -10.08849557519999962, 0.000000000000000000 ) ) ;
#6823=DIRECTION ( 'NONE',  ( 0.4794255386042041156, 0.000000000000000000, 0.8775825618903722036 ) ) ;
#6847=DIRECTION ( 'NONE',  ( 0.000000000000000000, 1.000000000000000000, 0.000000000000000000 ) ) ;
#6852=EDGE_CURVE ( 'NONE', #8881, #28111, #100, .T. ) ;
#6855=EDGE_LOOP ( 'NONE', ( #25803, #25733, #25623, #8165 ) ) ;
#6859=DIRECTION ( 'NONE',  ( 0.4794255386042000078, 0.000000000000000000, 0.8775825618903743131 ) ) ;
#6862=CIRCLE ( 'NONE', #5477, 0.3500000000000003664 ) ;
#6868=CARTESIAN_POINT ( 'NONE',  ( 0.000000000000000000, -11.50000000000000000, 0.000000000000000000 ) ) ;
#6874=DIRECTION ( 'NONE',  ( 0.000000000000000000, 1.000000000000000000, 0.000000000000000000 ) ) ;
#6877=AXIS2_PLACEMENT_3D ( 'NONE', #23147, #27233, #23010 ) ;
#6883=EDGE_CURVE ( 'NONE', #20553, #17731, #1060, .T. ) ;
#6886=DIRECTION ( 'NONE',  ( 0.000000000000000000, 1.000000000000000000, 0.000000000000000000 ) ) ;
#6889=TOROIDAL_SURFACE ( 'NONE', #11033, 14.25000000000000000, 2.000000000000000000 ) ;
#6890=DIRECTION ( 'NONE',  ( 0.8775825618903722036, 0.000000000000000000, -0.4794255386042041156 ) ) ;
#6892=EDGE_CURVE ( 'NONE', #4674, #20739, #4226, .T. ) ;
#6902=AXIS2_PLACEMENT_3D ( 'NONE', #17323, #26502, #24168 ) ;
#6921=ORIENTED_EDGE ( 'NONE', *, *, #24301, .T. ) ;
#6932=DIRECTION ( 'NONE',  ( 0.000000000000000000, 1.000000000000000000, 0.000000000000000000 ) ) ;
#6943=AXIS2_PLACEMENT_3D ( 'NONE', #3035, #20799, #27502 ) ;
#6946=CARTESIAN_POINT ( 'NONE',  ( 0.000000000000000000, -38.34400911419999858, 0.000000000000000000 ) ) ;
#6947=TOROIDAL_SURFACE ( 'NONE', #1386, 60.66666666670000296, 10.00000000000000000 ) ;
#6950=DIRECTION ( 'NONE',  ( 1.000000000000000000, 0.000000000000000000, 0.000000000000000000 ) ) ;
#6954=ORIENTED_EDGE ( 'NONE', *, *, #24072, .F. ) ;
#6970=ORIENTED_EDGE ( 'NONE', *, *, #15368, .F. ) ;
#6971=EDGE_LOOP ( 'NONE', ( #4972, #14678, #12232, #23322 ) ) ;
#6980=FACE_OUTER_BOUND ( 'NONE', #15337, .T. ) ;
#6989=CARTESIAN_POINT ( 'NONE',  ( 10.35605037799999906, -12.64149019679999952, 18.95662306240000206 ) ) ;
#6995=ADVANCED_FACE ( 'NONE', ( #5071 ), #21793, .F. ) ;
#7001=CIRCLE ( 'NONE', #2359, 1.999999999999999556 ) ;
#7003=AXIS2_PLACEMENT_3D ( 'NONE', #24233, #6014, #23944 ) ;
#7006=ORIENTED_EDGE ( 'NONE', *, *, #25539, .T. ) ;
#7019=EDGE_LOOP ( 'NONE', ( #13028, #18071, #12083, #7632 ) ) ;
#7024=EDGE_CURVE ( 'NONE', #5596, #28180, #11559, .T. ) ;
#7031=LINE ( 'NONE', #11516, #9538 ) ;
#7032=AXIS2_PLACEMENT_3D ( 'NONE', #4327, #8391, #2150 ) ;
#7035=CARTESIAN_POINT ( 'NONE',  ( 27.68682485439999752, -24.50000000000000000, 50.68039294919999804 ) ) ;
#7036=CARTESIAN_POINT ( 'NONE',  ( 0.000000000000000000, -26.29689110869999880, 0.000000000000000000 ) ) ;
#7048=TOROIDAL_SURFACE ( 'NONE', #8863, 24.50000000000000000, 3.000000000000000000 ) ;
#7058=DIRECTION ( 'NONE',  ( 1.000000000000000000, 0.000000000000000000, 0.000000000000000000 ) ) ;
#7063=DIRECTION ( 'NONE',  ( 0.4794255386042041156, 0.000000000000000000, 0.8775825618903722036 ) ) ;
#7072=CONICAL_SURFACE ( 'NONE', #14025, 53.75557630319999447, 1.380808038880000144 ) ;
#7092=ORIENTED_EDGE ( 'NONE', *, *, #22845, .F. ) ;
#7110=AXIS2_PLACEMENT_3D ( 'NONE', #6795, #10834, #2134 ) ;
#7119=FACE_OUTER_BOUND ( 'NONE', #10241, .T. ) ;
#7124=AXIS2_PLACEMENT_3D ( 'NONE', #25338, #436, #9430 ) ;
#7126=DIRECTION ( 'NONE',  ( 0.4794255386042041156, 0.000000000000000000, 0.8775825618903722036 ) ) ;
#7149=AXIS2_PLACEMENT_3D ( 'NONE', #8239, #23835, #18913 ) ;
#7159=CARTESIAN_POINT ( 'NONE',  ( 31.00000000000000000, -11.00000000000000000, 4.500000000000000000 ) ) ;
#7161=EDGE_CURVE ( 'NONE', #5109, #914, #16065, .T. ) ;
#7162=AXIS2_PLACEMENT_3D ( 'NONE', #10622, #26257, #9727 ) ;
#7176=CARTESIAN_POINT ( 'NONE',  ( 29.17304402409999753, -40.00000000000000000, 53.40089889099999709 ) ) ;
#7177=DIRECTION ( 'NONE',  ( -0.3390050494208429743, 0.7071067811866730279, -0.6205445805637129775 ) ) ;
#7222=DIRECTION ( 'NONE',  ( 0.4794255386042040601, 0.000000000000000000, 0.8775825618903720926 ) ) ;
#7231=CARTESIAN_POINT ( 'NONE',  ( 0.000000000000000000, -11.55246854740000018, 0.000000000000000000 ) ) ;
#7235=LINE ( 'NONE', #20484, #6236 ) ;
#7238=DIRECTION ( 'NONE',  ( 0.4794255386042033384, 0.000000000000000000, 0.8775825618903726477 ) ) ;
#7245=CARTESIAN_POINT ( 'NONE',  ( 4.500000000000000000, -15.00000000000000000, -40.50000000000000000 ) ) ;
#7252=ORIENTED_EDGE ( 'NONE', *, *, #26009, .F. ) ;
#7288=ADVANCED_FACE ( 'NONE', ( #28008 ), #10343, .T. ) ;
#7298=ORIENTED_EDGE ( 'NONE', *, *, #13312, .F. ) ;
#7304=ORIENTED_EDGE ( 'NONE', *, *, #26378, .F. ) ;
#7307=CARTESIAN_POINT ( 'NONE',  ( 0.000000000000000000, -24.50000000000000000, 0.000000000000000000 ) ) ;
#7309=ORIENTED_EDGE ( 'NONE', *, *, #6892, .T. ) ;
#7315=CARTESIAN_POINT ( 'NONE',  ( 0.000000000000000000, -25.10000000000000142, 0.000000000000000000 ) ) ;
#7323=DIRECTION ( 'NONE',  ( 0.000000000000000000, -1.000000000000000000, 0.000000000000000000 ) ) ;
#7343=ORIENTED_EDGE ( 'NONE', *, *, #1377, .T. ) ;
#7346=EDGE_CURVE ( 'NONE', #11658, #14280, #12673, .T. ) ;
#7356=AXIS2_PLACEMENT_3D ( 'NONE', #5833, #23604, #10046 ) ;
#7357=DIRECTION ( 'NONE',  ( 0.000000000000000000, 1.000000000000000000, 0.000000000000000000 ) ) ;
#7365=CIRCLE ( 'NONE', #5503, 55.50192378860000275 ) ;
#7380=VERTEX_POINT ( 'NONE', #12812 ) ;
#7387=VECTOR ( 'NONE', #13078, 1000.000000000000114 ) ;
#7389=DIRECTION ( 'NONE',  ( 0.4794255386042036715, 0.000000000000000000, 0.8775825618903723147 ) ) ;
#7395=DIRECTION ( 'NONE',  ( 0.000000000000000000, 1.000000000000000000, 0.000000000000000000 ) ) ;
#7433=EDGE_CURVE ( 'NONE', #12945, #22875, #27419, .T. ) ;
#7435=CIRCLE ( 'NONE', #27882, 2.999999999999998224 ) ;
#7437=AXIS2_PLACEMENT_3D ( 'NONE', #18156, #6649, #15512 ) ;
#7441=DIRECTION ( 'NONE',  ( 0.000000000000000000, 1.000000000000000000, 0.000000000000000000 ) ) ;
#7453=ORIENTED_EDGE ( 'NONE', *, *, #3942, .T. ) ;
#7472=FACE_OUTER_BOUND ( 'NONE', #1599, .T. ) ;
#7474=DIRECTION ( 'NONE',  ( 0.000000000000000000, -1.000000000000000000, 0.000000000000000000 ) ) ;
#7475=DIRECTION ( 'NONE',  ( 0.000000000000000000, 1.000000000000000000, 0.000000000000000000 ) ) ;
#7493=DIRECTION ( 'NONE',  ( 0.4794255386042000078, 0.000000000000000000, 0.8775825618903743131 ) ) ;
#7498=CIRCLE ( 'NONE', #23751, 0.4999999999999981126 ) ;
#7501=VECTOR ( 'NONE', #474, 1000.000000000000000 ) ;
#7529=CIRCLE ( 'NONE', #14918, 55.50192378860000275 ) ;
#7539=VERTEX_POINT ( 'NONE', #5543 ) ;
#7548=AXIS2_PLACEMENT_3D ( 'NONE', #318, #26370, #9158 ) ;
#7551=ORIENTED_EDGE ( 'NONE', *, *, #13517, .T. ) ;
#7557=ORIENTED_EDGE ( 'NONE', *, *, #14502, .T. ) ;
#7560=EDGE_CURVE ( 'NONE', #2039, #11046, #13425, .T. ) ;
#7575=DIRECTION ( 'NONE',  ( 0.4151946956541399669, 0.5000000000001689759, 0.7600087925152558821 ) ) ;
#7581=ORIENTED_EDGE ( 'NONE', *, *, #429, .F. ) ;
#7583=AXIS2_PLACEMENT_3D ( 'NONE', #1621, #26075, #1750 ) ;
#7586=ORIENTED_EDGE ( 'NONE', *, *, #20330, .F. ) ;
#7592=ORIENTED_EDGE ( 'NONE', *, *, #3612, .T. ) ;
#7616=CARTESIAN_POINT ( 'NONE',  ( 0.000000000000000000, -16.10310889129999623, 0.000000000000000000 ) ) ;
#7619=ORIENTED_EDGE ( 'NONE', *, *, #7841, .F. ) ;
#7620=CONICAL_SURFACE ( 'NONE', #22016, 53.75557630319999447, 1.380808038880000144 ) ;
#7627=CARTESIAN_POINT ( 'NONE',  ( 0.000000000000000000, -26.29689110869999880, 0.000000000000000000 ) ) ;
#7632=ORIENTED_EDGE ( 'NONE', *, *, #26451, .F. ) ;
#7653=CARTESIAN_POINT ( 'NONE',  ( 0.000000000000000000, -15.49681045920000066, 0.000000000000000000 ) ) ;
#7654=CARTESIAN_POINT ( 'NONE',  ( -4.500000000000000000, -13.00000000000000000, 50.00000000000000000 ) ) ;
#7661=DIRECTION ( 'NONE',  ( 1.000000000000000000, 0.000000000000000000, 0.000000000000000000 ) ) ;
#7667=VECTOR ( 'NONE', #8701, 1000.000000000000114 ) ;
#7668=EDGE_CURVE ( 'NONE', #15688, #27211, #21734, .T. ) ;
#7673=EDGE_CURVE ( 'NONE', #7380, #20895, #17095, .T. ) ;
#7689=DIRECTION ( 'NONE',  ( 0.000000000000000000, 0.000000000000000000, -1.000000000000000000 ) ) ;
#7692=DIRECTION ( 'NONE',  ( 0.4794255386042040046, 0.000000000000000000, 0.8775825618903722036 ) ) ;
#7700=CARTESIAN_POINT ( 'NONE',  ( 50.00000000000000000, -15.00000000000000000, 1.865174681369999824E-14 ) ) ;
#7714=ORIENTED_EDGE ( 'NONE', *, *, #7668, .F. ) ;
#7720=ORIENTED_EDGE ( 'NONE', *, *, #22928, .F. ) ;
#7727=DIRECTION ( 'NONE',  ( 1.000000000000000000, 0.000000000000000000, 0.000000000000000000 ) ) ;
#7730=ADVANCED_FACE ( 'NONE', ( #13222 ), #23149, .F. ) ;
#7752=DIRECTION ( 'NONE',  ( 0.000000000000000000, 1.000000000000000000, 0.000000000000000000 ) ) ;
#7756=CONICAL_SURFACE ( 'NONE', #26815, 55.67692378859999280, 1.047197551199999799 ) ;
#7761=DIRECTION ( 'NONE',  ( 0.000000000000000000, 1.000000000000000000, 0.000000000000000000 ) ) ;
#7766=EDGE_LOOP ( 'NONE', ( #15982, #19942, #20352, #27101 ) ) ;
#7769=ORIENTED_EDGE ( 'NONE', *, *, #19606, .T. ) ;
#7778=VERTEX_POINT ( 'NONE', #15695 ) ;
#7781=DIRECTION ( 'NONE',  ( 1.000000000000000000, 0.000000000000000000, 0.000000000000000000 ) ) ;
#7790=DIRECTION ( 'NONE',  ( 0.4794255386042041156, 0.000000000000000000, 0.8775825618903722036 ) ) ;
#7792=ADVANCED_FACE ( 'NONE', ( #13811 ), #6373, .F. ) ;
#7797=CARTESIAN_POINT ( 'NONE',  ( 26.77683864449999973, -33.79999999999999716, 49.01467436490000296 ) ) ;
#7822=ORIENTED_EDGE ( 'NONE', *, *, #16181, .T. ) ;
#7828=AXIS2_PLACEMENT_3D ( 'NONE', #13527, #27104, #4945 ) ;
#7841=EDGE_CURVE ( 'NONE', #731, #22563, #11915, .T. ) ;
#7844=ORIENTED_EDGE ( 'NONE', *, *, #6042, .F. ) ;
#7851=CARTESIAN_POINT ( 'NONE',  ( -50.00000000000000000, -11.00000000000000000, 4.500000000000000000 ) ) ;
#7852=CARTESIAN_POINT ( 'NONE',  ( 0.000000000000000000, -13.40000000000000036, 0.000000000000000000 ) ) ;
#7868=DIRECTION ( 'NONE',  ( 0.4794255386042000078, 0.000000000000000000, 0.8775825618903743131 ) ) ;
#7870=DIRECTION ( 'NONE',  ( 0.8775825618903722036, 0.000000000000000000, -0.4794255386042041156 ) ) ;
#7875=CIRCLE ( 'NONE', #15754, 55.50192378860000275 ) ;
#7882=ORIENTED_EDGE ( 'NONE', *, *, #18238, .F. ) ;
#7888=FACE_OUTER_BOUND ( 'NONE', #18880, .T. ) ;
#7894=DIRECTION ( 'NONE',  ( 0.4794255386042000078, 0.000000000000000000, 0.8775825618903743131 ) ) ;
#7914=ORIENTED_EDGE ( 'NONE', *, *, #26886, .T. ) ;
#7915=DIRECTION ( 'NONE',  ( 0.4151946956541399669, 0.5000000000001689759, 0.7600087925152558821 ) ) ;
#7934=AXIS2_PLACEMENT_3D ( 'NONE', #13101, #17349, #19388 ) ;
#7937=CYLINDRICAL_SURFACE ( 'NONE', #27996, 61.34999999999998721 ) ;
#7953=CARTESIAN_POINT ( 'NONE',  ( 0.000000000000000000, -10.95575221240000019, 0.000000000000000000 ) ) ;
#7963=LINE ( 'NONE', #25745, #4066 ) ;
#7968=DIRECTION ( 'NONE',  ( 1.000000000000000000, 0.000000000000000000, 3.652049423109066841E-16 ) ) ;
#7974=EDGE_CURVE ( 'NONE', #11046, #2039, #13538, .T. ) ;
#7990=EDGE_LOOP ( 'NONE', ( #27218, #16604, #23206, #10724 ) ) ;
#7996=DIRECTION ( 'NONE',  ( -1.000000000000000000, 0.000000000000000000, 0.000000000000000000 ) ) ;
#8005=PLANE ( 'NONE',  #1104 ) ;
#8007=EDGE_CURVE ( 'NONE', #22875, #12945, #7529, .T. ) ;
#8019=DIRECTION ( 'NONE',  ( 0.4794255386042036715, 0.000000000000000000, 0.8775825618903724257 ) ) ;
#8030=EDGE_CURVE ( 'NONE', #20122, #8526, #20195, .T. ) ;
#8032=ADVANCED_FACE ( 'NONE', ( #6800, #24720, #26466, #15358, #19747, #2434 ), #2138, .T. ) ;
#8044=DIRECTION ( 'NONE',  ( 0.4794255386042040601, 0.000000000000000000, 0.8775825618903720926 ) ) ;
#8046=ORIENTED_EDGE ( 'NONE', *, *, #5733, .T. ) ;
#8047=DIRECTION ( 'NONE',  ( 1.000000000000000000, 0.000000000000000000, 0.000000000000000000 ) ) ;
#8050=DIRECTION ( 'NONE',  ( 0.4794255386042033384, 0.000000000000000000, 0.8775825618903726477 ) ) ;
#8051=ORIENTED_EDGE ( 'NONE', *, *, #5118, .T. ) ;
#8053=CIRCLE ( 'NONE', #25736, 59.33923303830000151 ) ;
#8054=AXIS2_PLACEMENT_3D ( 'NONE', #18776, #27672, #27227 ) ;
#8059=EDGE_CURVE ( 'NONE', #14426, #1856, #23776, .T. ) ;
#8081=ORIENTED_EDGE ( 'NONE', *, *, #19348, .T. ) ;
#8084=AXIS2_PLACEMENT_3D ( 'NONE', #28737, #6459, #26575 ) ;
#8094=EDGE_CURVE ( 'NONE', #3189, #23988, #268, .T. ) ;
#8097=ADVANCED_FACE ( 'NONE', ( #2282 ), #4312, .F. ) ;
#8098=AXIS2_PLACEMENT_3D ( 'NONE', #6182, #20832, #8223 ) ;
#8101=DIRECTION ( 'NONE',  ( 0.000000000000000000, 1.000000000000000000, 0.000000000000000000 ) ) ;
#8105=DIRECTION ( 'NONE',  ( -0.8775825618903722036, 0.000000000000000000, 0.4794255386042041156 ) ) ;
#8114=FACE_OUTER_BOUND ( 'NONE', #15441, .T. ) ;
#8117=DIRECTION ( 'NONE',  ( 1.000000000000000000, 0.000000000000000000, 0.000000000000000000 ) ) ;
#8123=EDGE_CURVE ( 'NONE', #7539, #77, #19953, .T. ) ;
#8137=AXIS2_PLACEMENT_3D ( 'NONE', #5959, #28121, #27584 ) ;
#8165=ORIENTED_EDGE ( 'NONE', *, *, #1947, .F. ) ;
#8175=ORIENTED_EDGE ( 'NONE', *, *, #11974, .T. ) ;
#8178=CIRCLE ( 'NONE', #17500, 22.39904313779999612 ) ;
#8189=VERTEX_POINT ( 'NONE', #8981 ) ;
#8191=CARTESIAN_POINT ( 'NONE',  ( -11.74592569580000045, -11.00000000000000000, -21.50077276629999901 ) ) ;
#8210=ORIENTED_EDGE ( 'NONE', *, *, #16324, .F. ) ;
#8211=DIRECTION ( 'NONE',  ( -0.01257738078990017563, -0.9996558222130138560, -0.02302274110720029660 ) ) ;
#8213=ORIENTED_EDGE ( 'NONE', *, *, #17200, .T. ) ;
#8223=DIRECTION ( 'NONE',  ( 1.000000000000000000, 0.000000000000000000, 0.000000000000000000 ) ) ;
#8224=EDGE_LOOP ( 'NONE', ( #18461, #14100 ) ) ;
#8236=VECTOR ( 'NONE', #3648, 1000.000000000000000 ) ;
#8239=CARTESIAN_POINT ( 'NONE',  ( 26.77683864449999973, -19.40000000000000213, 49.01467436490000296 ) ) ;
#8241=EDGE_CURVE ( 'NONE', #20661, #13365, #2299, .T. ) ;
#8246=CARTESIAN_POINT ( 'NONE',  ( 40.50000000000000000, -15.00000000000000000, 4.500000000000000000 ) ) ;
#8254=CARTESIAN_POINT ( 'NONE',  ( -1.865174681369999824E-14, -15.00000000000000000, 31.00000000000000000 ) ) ;
#8262=CONICAL_SURFACE ( 'NONE', #24570, 11.99999999999999822, 0.02623728384790100648 ) ;
#8267=DIRECTION ( 'NONE',  ( 0.000000000000000000, 1.000000000000000000, 0.000000000000000000 ) ) ;
#8271=EDGE_CURVE ( 'NONE', #8526, #4628, #721, .T. ) ;
#8286=DIRECTION ( 'NONE',  ( 0.4794255386042040046, 0.000000000000000000, 0.8775825618903722036 ) ) ;
#8310=CARTESIAN_POINT ( 'NONE',  ( 0.000000000000000000, -15.49681045920000066, 0.000000000000000000 ) ) ;
#8324=FACE_OUTER_BOUND ( 'NONE', #26506, .T. ) ;
#8326=AXIS2_PLACEMENT_3D ( 'NONE', #9904, #18948, #3365 ) ;
#8339=ORIENTED_EDGE ( 'NONE', *, *, #6852, .T. ) ;
#8343=ORIENTED_EDGE ( 'NONE', *, *, #8798, .T. ) ;
#8365=VERTEX_POINT ( 'NONE', #28197 ) ;
#8369=FACE_OUTER_BOUND ( 'NONE', #6079, .T. ) ;
#8377=AXIS2_PLACEMENT_3D ( 'NONE', #4808, #162, #9015 ) ;
#8382=DIRECTION ( 'NONE',  ( -6.123031769109999188E-17, 0.000000000000000000, 1.000000000000000000 ) ) ;
#8384=VERTEX_POINT ( 'NONE', #16990 ) ;
#8390=EDGE_CURVE ( 'NONE', #14401, #18033, #27902, .T. ) ;
#8391=DIRECTION ( 'NONE',  ( 0.000000000000000000, 1.000000000000000000, 0.000000000000000000 ) ) ;
#8397=LINE ( 'NONE', #1868, #25960 ) ;
#8399=ORIENTED_EDGE ( 'NONE', *, *, #17596, .T. ) ;
#8401=FACE_OUTER_BOUND ( 'NONE', #21697, .T. ) ;
#8413=EDGE_LOOP ( 'NONE', ( #19457, #1737, #3015, #25741 ) ) ;
#8421=LINE ( 'NONE', #19787, #7667 ) ;
#8427=EDGE_CURVE ( 'NONE', #2153, #2039, #4639, .T. ) ;
#8439=VERTEX_POINT ( 'NONE', #12866 ) ;
#8440=VECTOR ( 'NONE', #10338, 1000.000000000000000 ) ;
#8446=PLANE ( 'NONE',  #7934 ) ;
#8471=DIRECTION ( 'NONE',  ( 0.000000000000000000, 1.000000000000000000, 0.000000000000000000 ) ) ;
#8472=AXIS2_PLACEMENT_3D ( 'NONE', #20629, #25568, #16819 ) ;
#8474=ADVANCED_FACE ( 'NONE', ( #4444 ), #26168, .T. ) ;
#8483=ORIENTED_EDGE ( 'NONE', *, *, #5068, .F. ) ;
#8494=TOROIDAL_SURFACE ( 'NONE', #12227, 55.85192378860000417, 0.3499999999999999778 ) ;
#8496=DIRECTION ( 'NONE',  ( 0.8775825618903722036, 0.000000000000000000, -0.4794255386042041156 ) ) ;
#8510=FACE_BOUND ( 'NONE', #14683, .T. ) ;
#8511=ORIENTED_EDGE ( 'NONE', *, *, #27087, .F. ) ;
#8518=DIRECTION ( 'NONE',  ( 0.4794255386042040601, 0.000000000000000000, 0.8775825618903720926 ) ) ;
#8524=DIRECTION ( 'NONE',  ( 0.4794255386042040046, 0.000000000000000000, 0.8775825618903722036 ) ) ;
#8526=VERTEX_POINT ( 'NONE', #20631 ) ;
#8534=ORIENTED_EDGE ( 'NONE', *, *, #20740, .T. ) ;
#8567=CARTESIAN_POINT ( 'NONE',  ( 0.000000000000000000, -28.69999999999999929, 0.000000000000000000 ) ) ;
#8568=DIRECTION ( 'NONE',  ( 1.000000000000000000, 0.000000000000000000, 0.000000000000000000 ) ) ;
#8577=CARTESIAN_POINT ( 'NONE',  ( 0.000000000000000000, -2.000000000000000000, 0.000000000000000000 ) ) ;
#8584=DIRECTION ( 'NONE',  ( 1.224606353819999829E-16, 0.000000000000000000, -1.000000000000000000 ) ) ;
#8589=ORIENTED_EDGE ( 'NONE', *, *, #1377, .F. ) ;
#8590=CARTESIAN_POINT ( 'NONE',  ( 0.000000000000000000, -16.10310889129999623, 0.000000000000000000 ) ) ;
#8595=CARTESIAN_POINT ( 'NONE',  ( 0.000000000000000000, -2.000000000000000000, 0.000000000000000000 ) ) ;
#8651=ORIENTED_EDGE ( 'NONE', *, *, #23302, .T. ) ;
#8657=DIRECTION ( 'NONE',  ( 0.000000000000000000, 1.000000000000000000, 0.000000000000000000 ) ) ;
#8666=EDGE_CURVE ( 'NONE', #14011, #11658, #5112, .T. ) ;
#8701=DIRECTION ( 'NONE',  ( -0.4707989697561778542, 0.1888473936500709438, -0.8617917335343248109 ) ) ;
#8702=DIRECTION ( 'NONE',  ( -0.4151946956541399669, 0.5000000000001689759, -0.7600087925152558821 ) ) ;
#8705=FACE_OUTER_BOUND ( 'NONE', #16353, .T. ) ;
#8707=DIRECTION ( 'NONE',  ( 1.000000000000000000, 0.000000000000000000, 0.000000000000000000 ) ) ;
#8718=CARTESIAN_POINT ( 'NONE',  ( -4.500000000000000000, -13.00000000000000000, 31.00000000000000000 ) ) ;
#8721=LINE ( 'NONE', #2345, #3406 ) ;
#8732=ORIENTED_EDGE ( 'NONE', *, *, #28182, .F. ) ;
#8734=CARTESIAN_POINT ( 'NONE',  ( 0.000000000000000000, -15.00000000000000000, 0.000000000000000000 ) ) ;
#8737=FACE_OUTER_BOUND ( 'NONE', #18807, .T. ) ;
#8756=CIRCLE ( 'NONE', #12481, 61.35000000000000142 ) ;
#8772=DIRECTION ( 'NONE',  ( 0.8775825618903722036, 0.000000000000000000, -0.4794255386042041156 ) ) ;
#8782=DIRECTION ( 'NONE',  ( 0.4794255386042040046, 0.000000000000000000, 0.8775825618903722036 ) ) ;
#8791=ORIENTED_EDGE ( 'NONE', *, *, #23302, .F. ) ;
#8794=CIRCLE ( 'NONE', #5105, 57.75000000000000000 ) ;
#8798=EDGE_CURVE ( 'NONE', #9643, #17262, #12700, .T. ) ;
#8807=DIRECTION ( 'NONE',  ( 0.000000000000000000, 1.000000000000000000, 0.000000000000000000 ) ) ;
#8808=ORIENTED_EDGE ( 'NONE', *, *, #5385, .F. ) ;
#8811=DIRECTION ( 'NONE',  ( 0.000000000000000000, 0.000000000000000000, 1.000000000000000000 ) ) ;
#8816=DIRECTION ( 'NONE',  ( 0.000000000000000000, -1.000000000000000000, 0.000000000000000000 ) ) ;
#8826=CARTESIAN_POINT ( 'NONE',  ( 26.77683864449999973, -23.00000000000000000, 49.01467436490000296 ) ) ;
#8830=VERTEX_POINT ( 'NONE', #26278 ) ;
#8836=AXIS2_PLACEMENT_3D ( 'NONE', #22538, #20043, #26765 ) ;
#8839=AXIS2_PLACEMENT_3D ( 'NONE', #21475, #24374, #25988 ) ;
#8845=CARTESIAN_POINT ( 'NONE',  ( 0.000000000000000000, -33.49689110869999809, 0.000000000000000000 ) ) ;
#8851=LINE ( 'NONE', #10876, #7387 ) ;
#8861=VECTOR ( 'NONE', #433, 999.9999999999998863 ) ;
#8863=AXIS2_PLACEMENT_3D ( 'NONE', #2190, #19798, #6558 ) ;
#8864=PRODUCT_CONTEXT ( 'NONE', #17800, 'mechanical' ) ;
#8878=DIRECTION ( 'NONE',  ( 0.000000000000000000, 1.000000000000000000, 0.000000000000000000 ) ) ;
#8881=VERTEX_POINT ( 'NONE', #1801 ) ;
#8902=EDGE_CURVE ( 'NONE', #20652, #20862, #24164, .T. ) ;
#8903=ORIENTED_EDGE ( 'NONE', *, *, #27855, .F. ) ;
#8923=CARTESIAN_POINT ( 'NONE',  ( 0.000000000000000000, -38.34400911419999858, 0.000000000000000000 ) ) ;
#8926=ORIENTED_EDGE ( 'NONE', *, *, #6361, .F. ) ;
#8928=CONICAL_SURFACE ( 'NONE', #14532, 52.86371681419998936, 1.437659999240000097 ) ;
#8929=CARTESIAN_POINT ( 'NONE',  ( -27.68682485439999752, -24.80000000000000071, -50.68039294919999804 ) ) ;
#8934=DIRECTION ( 'NONE',  ( 0.4794255386042040601, 0.000000000000000000, 0.8775825618903720926 ) ) ;
#8950=DIRECTION ( 'NONE',  ( 1.000000000000000000, 0.000000000000000000, 0.000000000000000000 ) ) ;
#8952=ORIENTED_EDGE ( 'NONE', *, *, #15580, .T. ) ;
#8958=AXIS2_PLACEMENT_3D ( 'NONE', #14229, #27199, #7238 ) ;
#8963=ADVANCED_FACE ( 'NONE', ( #9789, #11970 ), #23618, .F. ) ;
#8964=CARTESIAN_POINT ( 'NONE',  ( 4.500000000000000000, -15.00000000000000000, 40.50000000000000000 ) ) ;
#8975=VERTEX_POINT ( 'NONE', #1348 ) ;
#8979=DIRECTION ( 'NONE',  ( 0.000000000000000000, 1.000000000000000000, 0.000000000000000000 ) ) ;
#8981=CARTESIAN_POINT ( 'NONE',  ( 28.31007805460000171, -40.00000000000000000, 51.82125027960000097 ) ) ;
#8984=EDGE_LOOP ( 'NONE', ( #13670, #24173, #14841, #22842 ) ) ;
#8992=ORIENTED_EDGE ( 'NONE', *, *, #27253, .F. ) ;
#9007=ADVANCED_FACE ( 'NONE', ( #21030 ), #24183, .F. ) ;
#9015=DIRECTION ( 'NONE',  ( 0.4794255386042036715, 0.000000000000000000, 0.8775825618903724257 ) ) ;
#9021=AXIS2_PLACEMENT_3D ( 'NONE', #14206, #18866, #3140 ) ;
#9036=ADVANCED_FACE ( 'NONE', ( #27998 ), #28379, .F. ) ;
#9039=EDGE_LOOP ( 'NONE', ( #5701, #12768, #770, #20697 ) ) ;
#9047=VECTOR ( 'NONE', #20764, 999.9999999999998863 ) ;
#9050=FACE_OUTER_BOUND ( 'NONE', #18799, .T. ) ;
#9063=DIRECTION ( 'NONE',  ( 0.000000000000000000, 1.000000000000000000, 0.000000000000000000 ) ) ;
#9064=EDGE_LOOP ( 'NONE', ( #8175, #15911 ) ) ;
#9076=ORIENTED_EDGE ( 'NONE', *, *, #14169, .F. ) ;
#9081=TOROIDAL_SURFACE ( 'NONE', #12343, 19.50000000000000000, 3.000000000000000000 ) ;
#9107=DIRECTION ( 'NONE',  ( 0.000000000000000000, -1.000000000000000000, 0.000000000000000000 ) ) ;
#9110=DIRECTION ( 'NONE',  ( 1.000000000000000000, 0.000000000000000000, 0.000000000000000000 ) ) ;
#9123=ORIENTED_EDGE ( 'NONE', *, *, #1753, .T. ) ;
#9137=DIRECTION ( 'NONE',  ( 0.000000000000000000, 1.000000000000000000, 0.000000000000000000 ) ) ;
#9140=DIRECTION ( 'NONE',  ( 1.000000000000000000, 0.000000000000000000, 0.000000000000000000 ) ) ;
#9149=ORIENTED_EDGE ( 'NONE', *, *, #14459, .F. ) ;
#9158=DIRECTION ( 'NONE',  ( 1.000000000000000000, 0.000000000000000000, 0.000000000000000000 ) ) ;
#9159=EDGE_CURVE ( 'NONE', #17829, #14525, #15796, .T. ) ;
#9160=ORIENTED_EDGE ( 'NONE', *, *, #1196, .T. ) ;
#9161=VECTOR ( 'NONE', #8211, 1000.000000000000000 ) ;
#9167=ORIENTED_EDGE ( 'NONE', *, *, #19606, .F. ) ;
#9171=CIRCLE ( 'NONE', #7356, 10.00000000000000000 ) ;
#9175=DIRECTION ( 'NONE',  ( 0.000000000000000000, 1.000000000000000000, 0.000000000000000000 ) ) ;
#9195=EDGE_CURVE ( 'NONE', #2845, #4012, #9781, .T. ) ;
#9233=DIRECTION ( 'NONE',  ( 1.000000000000000000, 0.000000000000000000, 0.000000000000000000 ) ) ;
#9250=AXIS2_PLACEMENT_3D ( 'NONE', #18043, #15694, #7126 ) ;
#9252=CARTESIAN_POINT ( 'NONE',  ( -4.500000000000000000, -12.50000000000000000, -40.50000000000000000 ) ) ;
#9262=ORIENTED_EDGE ( 'NONE', *, *, #13652, .F. ) ;
#9268=EDGE_LOOP ( 'NONE', ( #18120, #21821 ) ) ;
#9271=ORIENTED_EDGE ( 'NONE', *, *, #8094, .F. ) ;
#9273=AXIS2_PLACEMENT_3D ( 'NONE', #8734, #17651, #24646 ) ;
#9297=ORIENTED_EDGE ( 'NONE', *, *, #26606, .T. ) ;
#9311=CIRCLE ( 'NONE', #9796, 55.67692378859999991 ) ;
#9317=EDGE_LOOP ( 'NONE', ( #13127, #22671, #13592, #28098 ) ) ;
#9328=DIRECTION ( 'NONE',  ( 0.000000000000000000, 1.000000000000000000, 0.000000000000000000 ) ) ;
#9338=AXIS2_PLACEMENT_3D ( 'NONE', #10741, #17338, #12935 ) ;
#9340=DIRECTION ( 'NONE',  ( 0.000000000000000000, -1.000000000000000000, 0.000000000000000000 ) ) ;
#9342=CARTESIAN_POINT ( 'NONE',  ( 0.000000000000000000, -15.49681045920000066, 0.000000000000000000 ) ) ;
#9343=DIRECTION ( 'NONE',  ( 0.000000000000000000, -1.000000000000000000, 0.000000000000000000 ) ) ;
#9347=ADVANCED_FACE ( 'NONE', ( #18073 ), #14424, .F. ) ;
#9350=ORIENTED_EDGE ( 'NONE', *, *, #6786, .F. ) ;
#9359=AXIS2_PLACEMENT_3D ( 'NONE', #22911, #20267, #2948 ) ;
#9366=ORIENTED_EDGE ( 'NONE', *, *, #28067, .T. ) ;
#9373=LINE ( 'NONE', #7654, #6571 ) ;
#9377=EDGE_CURVE ( 'NONE', #3841, #11046, #16287, .T. ) ;
#9393=VERTEX_POINT ( 'NONE', #17931 ) ;
#9397=CIRCLE ( 'NONE', #28483, 5.000000000000000000 ) ;
#9400=CARTESIAN_POINT ( 'NONE',  ( 0.000000000000000000, -10.00000000000000000, 0.000000000000000000 ) ) ;
#9405=FACE_OUTER_BOUND ( 'NONE', #23408, .T. ) ;
#9408=ORIENTED_EDGE ( 'NONE', *, *, #28165, .F. ) ;
#9419=DIRECTION ( 'NONE',  ( 0.000000000000000000, 1.000000000000000000, 0.000000000000000000 ) ) ;
#9422=CARTESIAN_POINT ( 'NONE',  ( 28.54979082390000045, -12.59999999999999964, 52.26004156059999417 ) ) ;
#9426=DIRECTION ( 'NONE',  ( 0.000000000000000000, 1.000000000000000000, 0.000000000000000000 ) ) ;
#9430=DIRECTION ( 'NONE',  ( 1.000000000000000000, 0.000000000000000000, 1.224606353819999829E-16 ) ) ;
#9433=VECTOR ( 'NONE', #27524, 999.9999999999998863 ) ;
#9435=TOROIDAL_SURFACE ( 'NONE', #21543, 52.35000000000000142, 1.000000000000000000 ) ;
#9458=PRODUCT_DEFINITION_CONTEXT ( 'detailed design', #16864, 'design' ) ;
#9462=DIRECTION ( 'NONE',  ( 0.000000000000000000, 1.000000000000000000, 0.000000000000000000 ) ) ;
#9474=CARTESIAN_POINT ( 'NONE',  ( 29.41275679339999982, -39.50000000000000000, 53.83969017199999740 ) ) ;
#9477=CARTESIAN_POINT ( 'NONE',  ( -4.500000000000000000, -13.00000000000000000, -31.00000000000000000 ) ) ;
#9484=ORIENTED_EDGE ( 'NONE', *, *, #6748, .T. ) ;
#9485=AXIS2_PLACEMENT_3D ( 'NONE', #8964, #408, #4900 ) ;
#9503=DIRECTION ( 'NONE',  ( 1.000000000000000000, 0.000000000000000000, 0.000000000000000000 ) ) ;
#9509=AXIS2_PLACEMENT_3D ( 'NONE', #20354, #10991, #27215 ) ;
#9523=FACE_OUTER_BOUND ( 'NONE', #1412, .T. ) ;
#9528=DIRECTION ( 'NONE',  ( 0.4151946956541399669, 0.5000000000001689759, 0.7600087925152558821 ) ) ;
#9538=VECTOR ( 'NONE', #9340, 1000.000000000000000 ) ;
#9554=FACE_OUTER_BOUND ( 'NONE', #1336, .T. ) ;
#9579=ORIENTED_EDGE ( 'NONE', *, *, #10688, .T. ) ;
#9617=ADVANCED_FACE ( 'NONE', ( #19424 ), #18169, .T. ) ;
#9619=CARTESIAN_POINT ( 'NONE',  ( 0.000000000000000000, -10.00000000000000000, 0.000000000000000000 ) ) ;
#9621=DIRECTION ( 'NONE',  ( 0.000000000000000000, 1.000000000000000000, 0.000000000000000000 ) ) ;
#9626=ORIENTED_EDGE ( 'NONE', *, *, #18472, .F. ) ;
#9629=EDGE_LOOP ( 'NONE', ( #10118, #1201, #10272, #10829 ) ) ;
#9632=CARTESIAN_POINT ( 'NONE',  ( 0.000000000000000000, -29.89689110870000022, 0.000000000000000000 ) ) ;
#9633=DIRECTION ( 'NONE',  ( 0.000000000000000000, 1.000000000000000000, 0.000000000000000000 ) ) ;
#9634=DIRECTION ( 'NONE',  ( 0.4794255386042040046, 0.000000000000000000, 0.8775825618903722036 ) ) ;
#9636=ORIENTED_EDGE ( 'NONE', *, *, #21671, .F. ) ;
#9637=EDGE_CURVE ( 'NONE', #22, #9643, #11162, .T. ) ;
#9643=VERTEX_POINT ( 'NONE', #4416 ) ;
#9665=VECTOR ( 'NONE', #27468, 1000.000000000000000 ) ;
#9672=AXIS2_PLACEMENT_3D ( 'NONE', #13837, #2780, #3083 ) ;
#9681=ORIENTED_EDGE ( 'NONE', *, *, #19249, .F. ) ;
#9682=CARTESIAN_POINT ( 'NONE',  ( -26.60903970598167589, -23.00000000000000000, -48.70752046822583736 ) ) ;
#9683=TOROIDAL_SURFACE ( 'NONE', #7828, 55.85192378860000417, 0.3499999999999999778 ) ;
#9696=CIRCLE ( 'NONE', #1339, 9.500000000000001776 ) ;
#9705=EDGE_CURVE ( 'NONE', #18448, #23053, #21881, .T. ) ;
#9706=ADVANCED_FACE ( 'NONE', ( #12841 ), #5154, .T. ) ;
#9710=ORIENTED_EDGE ( 'NONE', *, *, #9987, .T. ) ;
#9711=VECTOR ( 'NONE', #8816, 1000.000000000000000 ) ;
#9713=ORIENTED_EDGE ( 'NONE', *, *, #8007, .F. ) ;
#9719=LINE ( 'NONE', #3187, #6658 ) ;
#9727=DIRECTION ( 'NONE',  ( 0.4794255386042036715, 0.000000000000000000, 0.8775825618903724257 ) ) ;
#9735=AXIS2_PLACEMENT_3D ( 'NONE', #24541, #2560, #22363 ) ;
#9764=ORIENTED_EDGE ( 'NONE', *, *, #10665, .F. ) ;
#9767=CYLINDRICAL_SURFACE ( 'NONE', #23304, 9.500000000000001776 ) ;
#9771=DIRECTION ( 'NONE',  ( 1.000000000000000000, 0.000000000000000000, 0.000000000000000000 ) ) ;
#9781=CIRCLE ( 'NONE', #25149, 57.75000000000000000 ) ;
#9785=LINE ( 'NONE', #27437, #27034 ) ;
#9789=FACE_BOUND ( 'NONE', #9268, .T. ) ;
#9793=CARTESIAN_POINT ( 'NONE',  ( 0.000000000000000000, -30.50310889129999836, 0.000000000000000000 ) ) ;
#9796=AXIS2_PLACEMENT_3D ( 'NONE', #12070, #16597, #1180 ) ;
#9803=ORIENTED_EDGE ( 'NONE', *, *, #15191, .F. ) ;
#9805=LINE ( 'NONE', #18569, #28359 ) ;
#9807=DIRECTION ( 'NONE',  ( 0.000000000000000000, 1.000000000000000000, 0.000000000000000000 ) ) ;
#9812=ADVANCED_FACE ( 'NONE', ( #513 ), #20988, .F. ) ;
#9828=ADVANCED_FACE ( 'NONE', ( #218 ), #44, .T. ) ;
#9829=LINE ( 'NONE', #2712, #16815 ) ;
#9834=EDGE_LOOP ( 'NONE', ( #6584, #25737, #19048, #15202 ) ) ;
#9841=FACE_OUTER_BOUND ( 'NONE', #19896, .T. ) ;
#9842=CONICAL_SURFACE ( 'NONE', #12167, 55.67692378859999280, 1.047197551199999799 ) ;
#9849=DIRECTION ( 'NONE',  ( 0.000000000000000000, 1.000000000000000000, 0.000000000000000000 ) ) ;
#9851=VERTEX_POINT ( 'NONE', #3262 ) ;
#9854=AXIS2_PLACEMENT_3D ( 'NONE', #9864, #15988, #12047 ) ;
#9857=DIRECTION ( 'NONE',  ( 0.01257738078990017563, -0.9996558222130138560, 0.02302274110720029660 ) ) ;
#9859=ADVANCED_FACE ( 'NONE', ( #25268, #3532 ), #22938, .T. ) ;
#9863=VERTEX_POINT ( 'NONE', #16928 ) ;
#9864=CARTESIAN_POINT ( 'NONE',  ( 0.000000000000000000, -2.000000000000000000, 0.000000000000000000 ) ) ;
#9875=ORIENTED_EDGE ( 'NONE', *, *, #18999, .T. ) ;
#9880=ORIENTED_EDGE ( 'NONE', *, *, #28165, .T. ) ;
#9891=VECTOR ( 'NONE', #7727, 1000.000000000000000 ) ;
#9892=VECTOR ( 'NONE', #25375, 1000.000000000000000 ) ;
#9903=EDGE_CURVE ( 'NONE', #22563, #4998, #2364, .T. ) ;
#9904=CARTESIAN_POINT ( 'NONE',  ( 0.000000000000000000, -19.09689110869999951, 0.000000000000000000 ) ) ;
#9910=CARTESIAN_POINT ( 'NONE',  ( 0.000000000000000000, -2.000000000000000000, 0.000000000000000000 ) ) ;
#9923=ORIENTED_EDGE ( 'NONE', *, *, #10481, .T. ) ;
#9934=FACE_OUTER_BOUND ( 'NONE', #16971, .T. ) ;
#9949=AXIS2_PLACEMENT_3D ( 'NONE', #18060, #6847, #11629 ) ;
#9959=CARTESIAN_POINT ( 'NONE',  ( 4.500000000000000000, -12.50000000000000000, 50.00000000000000000 ) ) ;
#9964=EDGE_CURVE ( 'NONE', #3752, #5075, #19105, .T. ) ;
#9984=CARTESIAN_POINT ( 'NONE',  ( -10.73867332049999845, -11.85850980319999870, -19.65700966069999822 ) ) ;
#9987=EDGE_CURVE ( 'NONE', #12325, #11391, #6532, .T. ) ;
#9988=AXIS2_PLACEMENT_3D ( 'NONE', #3413, #1110, #21459 ) ;
#9989=ORIENTED_EDGE ( 'NONE', *, *, #22620, .T. ) ;
#9990=LINE ( 'NONE', #863, #20702 ) ;
#10000=ADVANCED_FACE ( 'NONE', ( #23763, #1637 ), #8446, .T. ) ;
#10012=FACE_BOUND ( 'NONE', #22202, .T. ) ;
#10020=EDGE_LOOP ( 'NONE', ( #16738, #3656, #21072, #15656 ) ) ;
#10041=AXIS2_PLACEMENT_3D ( 'NONE', #13011, #21922, #28614 ) ;
#10046=DIRECTION ( 'NONE',  ( 0.4794255386042042266, 0.000000000000000000, 0.8775825618903720926 ) ) ;
#10070=LINE ( 'NONE', #12533, #15361 ) ;
#10099=CIRCLE ( 'NONE', #20828, 9.499999999999998224 ) ;
#10100=CARTESIAN_POINT ( 'NONE',  ( 0.000000000000000000, -2.000000000000000000, 0.000000000000000000 ) ) ;
#10114=EDGE_CURVE ( 'NONE', #4043, #9863, #24698, .T. ) ;
#10118=ORIENTED_EDGE ( 'NONE', *, *, #16884, .T. ) ;
#10120=EDGE_CURVE ( 'NONE', #26131, #519, #4665, .T. ) ;
#10133=CIRCLE ( 'NONE', #13882, 0.3500000000000003664 ) ;
#10147=LINE ( 'NONE', #27544, #26544 ) ;
#10152=AXIS2_PLACEMENT_3D ( 'NONE', #17292, #26032, #19465 ) ;
#10153=AXIS2_PLACEMENT_3D ( 'NONE', #25340, #25037, #2753 ) ;
#10156=ORIENTED_EDGE ( 'NONE', *, *, #6786, .T. ) ;
#10179=DIRECTION ( 'NONE',  ( 0.4794255386042036715, 0.000000000000000000, 0.8775825618903724257 ) ) ;
#10182=CARTESIAN_POINT ( 'NONE',  ( 25.02601311510000315, -11.00000000000000000, 45.80980973070000317 ) ) ;
#10226=ORIENTED_EDGE ( 'NONE', *, *, #7346, .T. ) ;
#10234=CARTESIAN_POINT ( 'NONE',  ( -28.07036528529999941, -39.50000000000000000, -51.38245899869999533 ) ) ;
#10241=EDGE_LOOP ( 'NONE', ( #14140, #15157, #25095, #9167 ) ) ;
#10242=ADVANCED_FACE ( 'NONE', ( #24296 ), #19912, .F. ) ;
#10252=CARTESIAN_POINT ( 'NONE',  ( -26.77683864449999973, -26.59999999999999787, -49.01467436490000296 ) ) ;
#10256=AXIS2_PLACEMENT_3D ( 'NONE', #18011, #26909, #6950 ) ;
#10272=ORIENTED_EDGE ( 'NONE', *, *, #18902, .F. ) ;
#10273=EDGE_CURVE ( 'NONE', #28503, #22334, #6074, .T. ) ;
#10288=CARTESIAN_POINT ( 'NONE',  ( -4.500000000000000000, -15.00000000000000000, 31.00000000000000000 ) ) ;
#10297=CARTESIAN_POINT ( 'NONE',  ( 27.18988201479999844, -23.90155444570000043, 49.77074518290000071 ) ) ;
#10308=AXIS2_PLACEMENT_3D ( 'NONE', #26891, #2708, #7222 ) ;
#10309=DIRECTION ( 'NONE',  ( 0.000000000000000000, 1.000000000000000000, 0.000000000000000000 ) ) ;
#10310=ORIENTED_EDGE ( 'NONE', *, *, #5965, .F. ) ;
#10316=CARTESIAN_POINT ( 'NONE',  ( 26.60903970598167589, -30.20000000000000284, 48.70752046822583736 ) ) ;
#10319=DIRECTION ( 'NONE',  ( 1.000000000000000000, 0.000000000000000000, 1.278217298088173493E-15 ) ) ;
#10321=DIRECTION ( 'NONE',  ( 0.4794255386042041156, 0.000000000000000000, 0.8775825618903719816 ) ) ;
#10338=DIRECTION ( 'NONE',  ( 0.000000000000000000, -1.000000000000000000, 0.000000000000000000 ) ) ;
#10343=CYLINDRICAL_SURFACE ( 'NONE', #28324, 57.74999999999999289 ) ;
#10351=CIRCLE ( 'NONE', #3844, 55.67692378859999991 ) ;
#10356=ORIENTED_EDGE ( 'NONE', *, *, #10273, .T. ) ;
#10369=CARTESIAN_POINT ( 'NONE',  ( 25.02601311510000315, -6.000000000000000000, 45.80980973070000317 ) ) ;
#10370=EDGE_CURVE ( 'NONE', #54, #16026, #11903, .T. ) ;
#10372=ORIENTED_EDGE ( 'NONE', *, *, #6852, .F. ) ;
#10377=ORIENTED_EDGE ( 'NONE', *, *, #11307, .F. ) ;
#10378=CARTESIAN_POINT ( 'NONE',  ( 0.000000000000000000, -21.50000000000000000, 0.000000000000000000 ) ) ;
#10382=CARTESIAN_POINT ( 'NONE',  ( 11.74592569580000045, -14.00000000000000000, 21.50077276629999901 ) ) ;
#10390=DIRECTION ( 'NONE',  ( 0.000000000000000000, 1.000000000000000000, 0.000000000000000000 ) ) ;
#10419=CIRCLE ( 'NONE', #20207, 8.099999999999999645 ) ;
#10428=ADVANCED_FACE ( 'NONE', ( #6631 ), #3327, .F. ) ;
#10430=LINE ( 'NONE', #14816, #27821 ) ;
#10454=VERTEX_POINT ( 'NONE', #384 ) ;
#10464=PLANE ( 'NONE',  #22885 ) ;
#10478=DIRECTION ( 'NONE',  ( 0.000000000000000000, 1.000000000000000000, 0.000000000000000000 ) ) ;
#10481=EDGE_CURVE ( 'NONE', #20846, #27931, #5173, .T. ) ;
#10484=DIRECTION ( 'NONE',  ( -0.8775825618903722036, 0.000000000000000000, 0.4794255386042041156 ) ) ;
#10520=EDGE_CURVE ( 'NONE', #12535, #15620, #9785, .T. ) ;
#10536=ORIENTED_EDGE ( 'NONE', *, *, #22819, .F. ) ;
#10538=AXIS2_PLACEMENT_3D ( 'NONE', #21157, #25807, #8286 ) ;
#10541=EDGE_CURVE ( 'NONE', #28301, #15673, #13037, .T. ) ;
#10549=FACE_OUTER_BOUND ( 'NONE', #17666, .T. ) ;
#10557=AXIS2_PLACEMENT_3D ( 'NONE', #24508, #6886, #15751 ) ;
#10560=EDGE_LOOP ( 'NONE', ( #3679, #19871, #10687, #12831 ) ) ;
#10563=ORIENTED_EDGE ( 'NONE', *, *, #15947, .T. ) ;
#10586=EDGE_CURVE ( 'NONE', #23988, #25155, #15866, .T. ) ;
#10588=DIRECTION ( 'NONE',  ( 0.4794255386042036715, 0.000000000000000000, 0.8775825618903722036 ) ) ;
#10594=UNCERTAINTY_MEASURE_WITH_UNIT (LENGTH_MEASURE( 1.000000000000000082E-05 ), #1392, 'distance_accuracy_value', 'NONE');
#10595=FACE_OUTER_BOUND ( 'NONE', #19711, .T. ) ;
#10598=AXIS2_PLACEMENT_3D ( 'NONE', #7653, #14332, #20612 ) ;
#10608=ORIENTED_EDGE ( 'NONE', *, *, #6241, .F. ) ;
#10610=CARTESIAN_POINT ( 'NONE',  ( 0.000000000000000000, -2.000000000000000000, 0.000000000000000000 ) ) ;
#10622=CARTESIAN_POINT ( 'NONE',  ( 0.000000000000000000, -26.59999999999999787, 0.000000000000000000 ) ) ;
#10623=ADVANCED_FACE ( 'NONE', ( #10595 ), #19513, .F. ) ;
#10631=DIRECTION ( 'NONE',  ( 0.4794255386042000078, 0.000000000000000000, 0.8775825618903743131 ) ) ;
#10638=CIRCLE ( 'NONE', #25107, 60.85000000000000142 ) ;
#10652=VERTEX_POINT ( 'NONE', #22287 ) ;
#10655=ORIENTED_EDGE ( 'NONE', *, *, #8241, .F. ) ;
#10663=CARTESIAN_POINT ( 'NONE',  ( 0.000000000000000000, -23.30310889129999907, 0.000000000000000000 ) ) ;
#10664=EDGE_LOOP ( 'NONE', ( #1976, #9880, #26690, #764 ) ) ;
#10665=EDGE_CURVE ( 'NONE', #3189, #8384, #23306, .T. ) ;
#10687=ORIENTED_EDGE ( 'NONE', *, *, #18763, .F. ) ;
#10688=EDGE_CURVE ( 'NONE', #16942, #19419, #19587, .T. ) ;
#10697=EDGE_LOOP ( 'NONE', ( #4393, #9160, #26295, #20519 ) ) ;
#10698=CARTESIAN_POINT ( 'NONE',  ( -31.00000000000000000, -15.00000000000000000, 4.500000000000000000 ) ) ;
#10709=AXIS2_PLACEMENT_3D ( 'NONE', #25905, #21816, #23717 ) ;
#10710=ORIENTED_EDGE ( 'NONE', *, *, #12761, .T. ) ;
#10719=DIRECTION ( 'NONE',  ( -6.123031769109999188E-17, 0.000000000000000000, 1.000000000000000000 ) ) ;
#10724=ORIENTED_EDGE ( 'NONE', *, *, #8030, .F. ) ;
#10732=EDGE_LOOP ( 'NONE', ( #6970, #28346, #21430, #1075 ) ) ;
#10735=CARTESIAN_POINT ( 'NONE',  ( -4.500000000000000000, -12.50000000000000000, -50.00000000000000000 ) ) ;
#10741=CARTESIAN_POINT ( 'NONE',  ( 0.000000000000000000, -2.000000000000000000, 0.000000000000000000 ) ) ;
#10744=ADVANCED_FACE ( 'NONE', ( #21534 ), #2383, .F. ) ;
#10761=CARTESIAN_POINT ( 'NONE',  ( 0.000000000000000000, -2.000000000000000000, 0.000000000000000000 ) ) ;
#10762=DIRECTION ( 'NONE',  ( 0.4509255599460827435, -0.3396444637780623443, 0.8254137008871517134 ) ) ;
#10829=ORIENTED_EDGE ( 'NONE', *, *, #2197, .T. ) ;
#10834=DIRECTION ( 'NONE',  ( 0.000000000000000000, 1.000000000000000000, 0.000000000000000000 ) ) ;
#10839=CARTESIAN_POINT ( 'NONE',  ( 0.000000000000000000, -19.40000000000000213, 0.000000000000000000 ) ) ;
#10840=CARTESIAN_POINT ( 'NONE',  ( 26.69293917519999937, -29.89689110870000022, 48.86109741659999628 ) ) ;
#10847=ORIENTED_EDGE ( 'NONE', *, *, #21067, .T. ) ;
#10876=CARTESIAN_POINT ( 'NONE',  ( -11.78548194719999920, -15.31994771319999948, -21.57317999869999881 ) ) ;
#10884=CARTESIAN_POINT ( 'NONE',  ( 26.77683864449999973, -30.20000000000000284, 49.01467436490000296 ) ) ;
#10887=FACE_OUTER_BOUND ( 'NONE', #17402, .T. ) ;
#10888=AXIS2_PLACEMENT_3D ( 'NONE', #15290, #2216, #4249 ) ;
#10899=CARTESIAN_POINT ( 'NONE',  ( -25.77179612209999959, -37.57799544290000426, -47.17495636800000369 ) ) ;
#10901=AXIS2_PLACEMENT_3D ( 'NONE', #13352, #19769, #26631 ) ;
#10909=DIRECTION ( 'NONE',  ( 0.000000000000000000, 1.000000000000000000, 0.000000000000000000 ) ) ;
#10940=EDGE_LOOP ( 'NONE', ( #8339, #13940 ) ) ;
#10952=DIRECTION ( 'NONE',  ( 0.000000000000000000, 1.000000000000000000, 0.000000000000000000 ) ) ;
#10976=ADVANCED_FACE ( 'NONE', ( #6260 ), #10464, .T. ) ;
#10987=EDGE_CURVE ( 'NONE', #2039, #103, #28258, .T. ) ;
#10991=DIRECTION ( 'NONE',  ( 0.000000000000000000, 1.000000000000000000, 0.000000000000000000 ) ) ;
#11008=ORIENTED_EDGE ( 'NONE', *, *, #23610, .F. ) ;
#11009=ADVANCED_FACE ( 'NONE', ( #12939 ), #9842, .T. ) ;
#11013=CARTESIAN_POINT ( 'NONE',  ( 0.000000000000000000, -2.000000000000000000, 0.000000000000000000 ) ) ;
#11016=EDGE_CURVE ( 'NONE', #17262, #10454, #16920, .T. ) ;
#11017=DIRECTION ( 'NONE',  ( 0.000000000000000000, 1.000000000000000000, 0.000000000000000000 ) ) ;
#11019=VERTEX_POINT ( 'NONE', #24927 ) ;
#11023=FACE_OUTER_BOUND ( 'NONE', #6068, .T. ) ;
#11027=CARTESIAN_POINT ( 'NONE',  ( 0.000000000000000000, -29.89689110870000022, 0.000000000000000000 ) ) ;
#11029=VERTEX_POINT ( 'NONE', #22291 ) ;
#11033=AXIS2_PLACEMENT_3D ( 'NONE', #21992, #17622, #2041 ) ;
#11037=DIRECTION ( 'NONE',  ( 0.000000000000000000, -1.000000000000000000, 0.000000000000000000 ) ) ;
#11046=VERTEX_POINT ( 'NONE', #26821 ) ;
#11081=ORIENTED_EDGE ( 'NONE', *, *, #26858, .F. ) ;
#11088=VECTOR ( 'NONE', #22354, 1000.000000000000000 ) ;
#11098=CIRCLE ( 'NONE', #27443, 19.50000000000000000 ) ;
#11099=CARTESIAN_POINT ( 'NONE',  ( 0.000000000000000000, -22.69689110870000093, 0.000000000000000000 ) ) ;
#11102=DIRECTION ( 'NONE',  ( 0.000000000000000000, 1.000000000000000000, 0.000000000000000000 ) ) ;
#11113=AXIS2_PLACEMENT_3D ( 'NONE', #6192, #28482, #8518 ) ;
#11126=VERTEX_POINT ( 'NONE', #765 ) ;
#11129=DIRECTION ( 'NONE',  ( 0.000000000000000000, 1.000000000000000000, 0.000000000000000000 ) ) ;
#11135=CARTESIAN_POINT ( 'NONE',  ( -27.68682485439999752, -28.69999999999999929, -50.68039294919999804 ) ) ;
#11139=CIRCLE ( 'NONE', #14869, 55.50192378860000275 ) ;
#11144=DIRECTION ( 'NONE',  ( 0.000000000000000000, 1.000000000000000000, 0.000000000000000000 ) ) ;
#11154=VERTEX_POINT ( 'NONE', #18663 ) ;
#11159=AXIS2_PLACEMENT_3D ( 'NONE', #23027, #3078, #20838 ) ;
#11160=FACE_OUTER_BOUND ( 'NONE', #27702, .T. ) ;
#11162=CIRCLE ( 'NONE', #7003, 9.099999999999999645 ) ;
#11186=VECTOR ( 'NONE', #963, 1000.000000000000114 ) ;
#11190=AXIS2_PLACEMENT_3D ( 'NONE', #11288, #11129, #13479 ) ;
#11203=CARTESIAN_POINT ( 'NONE',  ( 0.000000000000000000, -39.50000000000000000, 0.000000000000000000 ) ) ;
#11205=FACE_OUTER_BOUND ( 'NONE', #20327, .T. ) ;
#11218=ORIENTED_EDGE ( 'NONE', *, *, #3466, .F. ) ;
#11229=CIRCLE ( 'NONE', #3362, 61.35000000000000142 ) ;
#11247=CARTESIAN_POINT ( 'NONE',  ( -26.89647983300000078, -10.52212389379999991, -49.23367609159999603 ) ) ;
#11248=ORIENTED_EDGE ( 'NONE', *, *, #28731, .F. ) ;
#11275=DIRECTION ( 'NONE',  ( 1.000000000000000000, 0.000000000000000000, 0.000000000000000000 ) ) ;
#11288=CARTESIAN_POINT ( 'NONE',  ( 0.000000000000000000, -37.57799544290000426, 0.000000000000000000 ) ) ;
#11300=DIRECTION ( 'NONE',  ( 1.000000000000000000, 0.000000000000000000, 0.000000000000000000 ) ) ;
#11307=EDGE_CURVE ( 'NONE', #8189, #26635, #16357, .T. ) ;
#11308=CARTESIAN_POINT ( 'NONE',  ( 0.000000000000000000, -2.000000000000000000, 0.000000000000000000 ) ) ;
#11316=DIRECTION ( 'NONE',  ( 0.000000000000000000, 1.000000000000000000, 0.000000000000000000 ) ) ;
#11322=CARTESIAN_POINT ( 'NONE',  ( 0.000000000000000000, -17.50000000000000000, 0.000000000000000000 ) ) ;
#11329=DIRECTION ( 'NONE',  ( 0.8775825618903722036, 0.000000000000000000, -0.4794255386042041156 ) ) ;
#11337=CARTESIAN_POINT ( 'NONE',  ( 6.831813925109999630, -13.50000000000000000, 12.50555150689999984 ) ) ;
#11343=AXIS2_PLACEMENT_3D ( 'NONE', #24652, #23060, #5128 ) ;
#11362=DIRECTION ( 'NONE',  ( 1.000000000000000000, 0.000000000000000000, 0.000000000000000000 ) ) ;
#11370=ORIENTED_EDGE ( 'NONE', *, *, #18031, .T. ) ;
#11373=VECTOR ( 'NONE', #25123, 1000.000000000000000 ) ;
#11376=DIRECTION ( 'NONE',  ( 0.4794255386042041156, 0.000000000000000000, 0.8775825618903720926 ) ) ;
#11377=CARTESIAN_POINT ( 'NONE',  ( 0.000000000000000000, -26.90310889129999694, 0.000000000000000000 ) ) ;
#11383=VECTOR ( 'NONE', #2784, 1000.000000000000000 ) ;
#11391=VERTEX_POINT ( 'NONE', #1699 ) ;
#11402=DIRECTION ( 'NONE',  ( 0.4794255386042040046, 0.000000000000000000, 0.8775825618903722036 ) ) ;
#11404=EDGE_CURVE ( 'NONE', #15395, #3254, #23797, .T. ) ;
#11405=CARTESIAN_POINT ( 'NONE',  ( 0.000000000000000000, -10.50000000000000000, 0.000000000000000000 ) ) ;
#11406=AXIS2_PLACEMENT_3D ( 'NONE', #15431, #481, #22160 ) ;
#11414=DIRECTION ( 'NONE',  ( 0.000000000000000000, 1.000000000000000000, 0.000000000000000000 ) ) ;
#11432=CARTESIAN_POINT ( 'NONE',  ( 0.000000000000000000, -15.49689110870000164, 0.000000000000000000 ) ) ;
#11451=EDGE_LOOP ( 'NONE', ( #3788, #1929, #25409, #18933 ) ) ;
#11454=CYLINDRICAL_SURFACE ( 'NONE', #5589, 9.500000000000001776 ) ;
#11467=EDGE_CURVE ( 'NONE', #22328, #16026, #9829, .T. ) ;
#11476=ORIENTED_EDGE ( 'NONE', *, *, #8390, .F. ) ;
#11481=DIRECTION ( 'NONE',  ( 0.4794255386042040601, 0.000000000000000000, 0.8775825618903720926 ) ) ;
#11482=ORIENTED_EDGE ( 'NONE', *, *, #13926, .T. ) ;
#11487=FACE_OUTER_BOUND ( 'NONE', #1194, .T. ) ;
#11503=EDGE_CURVE ( 'NONE', #3189, #2845, #5331, .T. ) ;
#11513=DIRECTION ( 'NONE',  ( 0.000000000000000000, 0.000000000000000000, 1.000000000000000000 ) ) ;
#11516=CARTESIAN_POINT ( 'NONE',  ( -27.68682485439999752, -24.80000000000000071, -50.68039294919999804 ) ) ;
#11520=DIRECTION ( 'NONE',  ( 0.000000000000000000, 1.000000000000000000, 0.000000000000000000 ) ) ;
#11524=ORIENTED_EDGE ( 'NONE', *, *, #26858, .T. ) ;
#11532=CARTESIAN_POINT ( 'NONE',  ( 0.000000000000000000, -37.08699221940000257, 0.000000000000000000 ) ) ;
#11534=CIRCLE ( 'NONE', #14368, 55.67692378859999991 ) ;
#11537=DIRECTION ( 'NONE',  ( 0.000000000000000000, 1.000000000000000000, 0.000000000000000000 ) ) ;
#11559=CIRCLE ( 'NONE', #10153, 22.39904313779999612 ) ;
#11568=CIRCLE ( 'NONE', #940, 0.3500000000000003664 ) ;
#11577=DIRECTION ( 'NONE',  ( 0.000000000000000000, 0.000000000000000000, 1.000000000000000000 ) ) ;
#11590=EDGE_LOOP ( 'NONE', ( #6360, #13430, #19441, #26953 ) ) ;
#11591=EDGE_CURVE ( 'NONE', #8975, #12823, #4258, .T. ) ;
#11592=AXIS2_PLACEMENT_3D ( 'NONE', #24801, #18088, #11513 ) ;
#11597=CARTESIAN_POINT ( 'NONE',  ( 0.000000000000000000, -13.40000000000000036, 0.000000000000000000 ) ) ;
#11625=ADVANCED_FACE ( 'NONE', ( #10887 ), #1497, .T. ) ;
#11629=DIRECTION ( 'NONE',  ( 1.000000000000000000, 0.000000000000000000, 0.000000000000000000 ) ) ;
#11638=CARTESIAN_POINT ( 'NONE',  ( 50.00000000000000000, -15.00000000000000000, 4.500000000000000000 ) ) ;
#11641=CIRCLE ( 'NONE', #23753, 55.67692378859999991 ) ;
#11646=ORIENTED_EDGE ( 'NONE', *, *, #19056, .F. ) ;
#11658=VERTEX_POINT ( 'NONE', #15566 ) ;
#11663=ORIENTED_EDGE ( 'NONE', *, *, #8666, .T. ) ;
#11664=AXIS2_PLACEMENT_3D ( 'NONE', #13872, #6890, #4406 ) ;
#11705=CIRCLE ( 'NONE', #23373, 6.999999999999997335 ) ;
#11712=EDGE_CURVE ( 'NONE', #23028, #13365, #27095, .T. ) ;
#11727=CIRCLE ( 'NONE', #19176, 12.00000000000000000 ) ;
#11749=EDGE_CURVE ( 'NONE', #8439, #18513, #1007, .T. ) ;
#11765=CONICAL_SURFACE ( 'NONE', #25280, 55.67692378859999280, 1.047197551199999799 ) ;
#11783=FACE_OUTER_BOUND ( 'NONE', #27605, .T. ) ;
#11791=CONICAL_SURFACE ( 'NONE', #18336, 55.67692378859999280, 1.047197551199999799 ) ;
#11795=CARTESIAN_POINT ( 'NONE',  ( -28.54979082390000045, -36.85000000000000142, -52.26004156059999417 ) ) ;
#11799=ORIENTED_EDGE ( 'NONE', *, *, #10520, .T. ) ;
#11811=DIRECTION ( 'NONE',  ( -0.8775825618903722036, 0.000000000000000000, 0.4794255386042041156 ) ) ;
#11826=VECTOR ( 'NONE', #25591, 999.9999999999998863 ) ;
#11830=EDGE_LOOP ( 'NONE', ( #26326, #19914 ) ) ;
#11847=EDGE_LOOP ( 'NONE', ( #1009, #14561, #484, #24013 ) ) ;
#11871=CARTESIAN_POINT ( 'NONE',  ( -26.69293917519999937, -22.69689110870000093, -48.86109741659999628 ) ) ;
#11894=AXIS2_PLACEMENT_3D ( 'NONE', #11203, #29, #15588 ) ;
#11902=DIRECTION ( 'NONE',  ( 0.000000000000000000, 1.000000000000000000, 0.000000000000000000 ) ) ;
#11903=LINE ( 'NONE', #2748, #8861 ) ;
#11915=LINE ( 'NONE', #27532, #17263 ) ;
#11930=LINE ( 'NONE', #18499, #21520 ) ;
#11936=ORIENTED_EDGE ( 'NONE', *, *, #9987, .F. ) ;
#11941=ORIENTED_EDGE ( 'NONE', *, *, #15580, .F. ) ;
#11958=DIRECTION ( 'NONE',  ( 0.000000000000000000, 1.000000000000000000, 0.000000000000000000 ) ) ;
#11962=DIRECTION ( 'NONE',  ( 0.4794255386042000078, 0.000000000000000000, 0.8775825618903743131 ) ) ;
#11965=EDGE_CURVE ( 'NONE', #519, #3448, #13760, .T. ) ;
#11970=FACE_OUTER_BOUND ( 'NONE', #12194, .T. ) ;
#11971=ORIENTED_EDGE ( 'NONE', *, *, #1196, .F. ) ;
#11974=EDGE_CURVE ( 'NONE', #16418, #21532, #19950, .T. ) ;
#11984=CARTESIAN_POINT ( 'NONE',  ( 26.60903970598167589, -33.79999999999999716, 48.70752046822583736 ) ) ;
#11994=CARTESIAN_POINT ( 'NONE',  ( -31.00000000000000000, -15.00000000000000000, -2.398081733189999864E-14 ) ) ;
#12001=AXIS2_PLACEMENT_3D ( 'NONE', #17422, #1985, #12734 ) ;
#12007=CARTESIAN_POINT ( 'NONE',  ( 0.000000000000000000, -36.20000000000000284, 0.000000000000000000 ) ) ;
#12014=DIRECTION ( 'NONE',  ( 0.4794255386042041711, 0.000000000000000000, 0.8775825618903720926 ) ) ;
#12021=CYLINDRICAL_SURFACE ( 'NONE', #23462, 58.55000000000003979 ) ;
#12023=CARTESIAN_POINT ( 'NONE',  ( 0.000000000000000000, -23.30310889129999907, 0.000000000000000000 ) ) ;
#12034=ADVANCED_FACE ( 'NONE', ( #11205 ), #17648, .T. ) ;
#12038=ORIENTED_EDGE ( 'NONE', *, *, #19596, .T. ) ;
#12047=DIRECTION ( 'NONE',  ( 0.4794255386042041156, 0.000000000000000000, 0.8775825618903722036 ) ) ;
#12053=ORIENTED_EDGE ( 'NONE', *, *, #27354, .F. ) ;
#12054=CYLINDRICAL_SURFACE ( 'NONE', #6488, 58.55000000000003979 ) ;
#12064=AXIS2_PLACEMENT_3D ( 'NONE', #4238, #15734, #15888 ) ;
#12067=DIRECTION ( 'NONE',  ( -0.4151946956541399669, 0.5000000000001689759, -0.7600087925152558821 ) ) ;
#12070=CARTESIAN_POINT ( 'NONE',  ( 0.000000000000000000, -26.90310889129999694, 0.000000000000000000 ) ) ;
#12075=DIRECTION ( 'NONE',  ( 0.4794255386042059475, 0.000000000000000000, 0.8775825618903710934 ) ) ;
#12083=ORIENTED_EDGE ( 'NONE', *, *, #19249, .T. ) ;
#12096=VERTEX_POINT ( 'NONE', #4672 ) ;
#12115=DIRECTION ( 'NONE',  ( 0.000000000000000000, -1.000000000000000000, 0.000000000000000000 ) ) ;
#12119=CIRCLE ( 'NONE', #4680, 55.50192378860000275 ) ;
#12125=EDGE_CURVE ( 'NONE', #12804, #14272, #13708, .T. ) ;
#12139=EDGE_CURVE ( 'NONE', #22328, #4674, #25106, .T. ) ;
#12148=DIRECTION ( 'NONE',  ( 0.000000000000000000, 1.000000000000000000, 0.000000000000000000 ) ) ;
#12150=DIRECTION ( 'NONE',  ( 0.000000000000000000, 1.000000000000000000, 0.000000000000000000 ) ) ;
#12152=LINE ( 'NONE', #21065, #16419 ) ;
#12160=MECHANICAL_DESIGN_GEOMETRIC_PRESENTATION_REPRESENTATION('',(#28040),#17276);
#12164=CARTESIAN_POINT ( 'NONE',  ( -25.57735248450000043, -26.54349610970000128, -46.81902967690000139 ) ) ;
#12165=DIRECTION ( 'NONE',  ( 0.000000000000000000, 0.000000000000000000, 1.000000000000000000 ) ) ;
#12167=AXIS2_PLACEMENT_3D ( 'NONE', #21853, #24186, #21431 ) ;
#12177=CIRCLE ( 'NONE', #28460, 55.67692378859999991 ) ;
#12186=CARTESIAN_POINT ( 'NONE',  ( 0.000000000000000000, -15.00000000000000000, 0.000000000000000000 ) ) ;
#12187=CYLINDRICAL_SURFACE ( 'NONE', #1373, 9.500000000000001776 ) ;
#12188=ORIENTED_EDGE ( 'NONE', *, *, #12139, .F. ) ;
#12194=EDGE_LOOP ( 'NONE', ( #25464, #18393 ) ) ;
#12208=EDGE_CURVE ( 'NONE', #15620, #1234, #26954, .T. ) ;
#12227=AXIS2_PLACEMENT_3D ( 'NONE', #19737, #8657, #19322 ) ;
#12230=DIRECTION ( 'NONE',  ( 0.000000000000000000, -1.000000000000000000, 0.000000000000000000 ) ) ;
#12232=ORIENTED_EDGE ( 'NONE', *, *, #21253, .F. ) ;
#12244=CARTESIAN_POINT ( 'NONE',  ( 0.000000000000000000, -25.10000000000000142, 0.000000000000000000 ) ) ;
#12263=CARTESIAN_POINT ( 'NONE',  ( 40.50000000000000000, -12.50000000000000000, 4.500000000000000000 ) ) ;
#12266=EDGE_LOOP ( 'NONE', ( #8399, #18285, #3490, #17054 ) ) ;
#12276=EDGE_CURVE ( 'NONE', #23028, #6664, #20930, .T. ) ;
#12296=LINE ( 'NONE', #16677, #21365 ) ;
#12306=TOROIDAL_SURFACE ( 'NONE', #17428, 60.66666666670000296, 10.00000000000000000 ) ;
#12307=DIRECTION ( 'NONE',  ( 0.000000000000000000, -1.000000000000000000, 0.000000000000000000 ) ) ;
#12317=EDGE_LOOP ( 'NONE', ( #22929, #2863, #18642, #12847 ) ) ;
#12322=CARTESIAN_POINT ( 'NONE',  ( 0.000000000000000000, -26.59999999999999787, 0.000000000000000000 ) ) ;
#12325=VERTEX_POINT ( 'NONE', #15242 ) ;
#12343=AXIS2_PLACEMENT_3D ( 'NONE', #15555, #24459, #152 ) ;
#12344=DIRECTION ( 'NONE',  ( 0.000000000000000000, 1.000000000000000000, 0.000000000000000000 ) ) ;
#12345=DIRECTION ( 'NONE',  ( 0.000000000000000000, 1.000000000000000000, 0.000000000000000000 ) ) ;
#12347=ORIENTED_EDGE ( 'NONE', *, *, #10987, .F. ) ;
#12352=ORIENTED_EDGE ( 'NONE', *, *, #27358, .F. ) ;
#12364=DIRECTION ( 'NONE',  ( 0.000000000000000000, 1.000000000000000000, 0.000000000000000000 ) ) ;
#12375=CARTESIAN_POINT ( 'NONE',  ( 4.500000000000000000, -11.00000000000000000, 40.50000000000000000 ) ) ;
#12381=ADVANCED_FACE ( 'NONE', ( #6980 ), #21364, .F. ) ;
#12389=EDGE_CURVE ( 'NONE', #27931, #19426, #7875, .T. ) ;
#12397=CARTESIAN_POINT ( 'NONE',  ( 27.68682485439999752, -17.89999999999999858, 50.68039294919999804 ) ) ;
#12398=ORIENTED_EDGE ( 'NONE', *, *, #1186, .F. ) ;
#12420=EDGE_CURVE ( 'NONE', #9643, #22, #5545, .T. ) ;
#12421=CIRCLE ( 'NONE', #28703, 61.35000000000000142 ) ;
#12428=AXIS2_PLACEMENT_3D ( 'NONE', #2042, #15256, #24468 ) ;
#12433=CARTESIAN_POINT ( 'NONE',  ( 27.18988201479999844, -29.29844555429999886, 49.77074518290000071 ) ) ;
#12441=ORIENTED_EDGE ( 'NONE', *, *, #14572, .T. ) ;
#12453=LINE ( 'NONE', #23135, #18619 ) ;
#12466=ORIENTED_EDGE ( 'NONE', *, *, #4107, .T. ) ;
#12478=AXIS2_PLACEMENT_3D ( 'NONE', #15183, #10952, #2118 ) ;
#12480=ADVANCED_FACE ( 'NONE', ( #23812 ), #27881, .T. ) ;
#12481=AXIS2_PLACEMENT_3D ( 'NONE', #16206, #13589, #810 ) ;
#12498=AXIS2_PLACEMENT_3D ( 'NONE', #11322, #4790, #22573 ) ;
#12507=EDGE_CURVE ( 'NONE', #17829, #1871, #5021, .T. ) ;
#12510=ORIENTED_EDGE ( 'NONE', *, *, #18989, .F. ) ;
#12513=DIRECTION ( 'NONE',  ( 1.000000000000000000, 0.000000000000000000, 0.000000000000000000 ) ) ;
#12519=EDGE_LOOP ( 'NONE', ( #8992, #16130, #19469, #21806 ) ) ;
#12533=CARTESIAN_POINT ( 'NONE',  ( 27.68682485439999752, -24.80000000000000071, 50.68039294919999804 ) ) ;
#12534=CARTESIAN_POINT ( 'NONE',  ( -27.68682485439999752, -25.10000000000000142, -50.68039294919999804 ) ) ;
#12535=VERTEX_POINT ( 'NONE', #10234 ) ;
#12538=LINE ( 'NONE', #19541, #22293 ) ;
#12540=AXIS2_PLACEMENT_3D ( 'NONE', #26973, #177, #20109 ) ;
#12559=TOROIDAL_SURFACE ( 'NONE', #16307, 55.85192378860000417, 0.3499999999999999778 ) ;
#12567=EDGE_LOOP ( 'NONE', ( #3907, #24496, #27242, #26882 ) ) ;
#12577=DIRECTION ( 'NONE',  ( 1.000000000000000000, 0.000000000000000000, 0.000000000000000000 ) ) ;
#12582=CIRCLE ( 'NONE', #6072, 9.500000000000001776 ) ;
#12585=AXIS2_PLACEMENT_3D ( 'NONE', #11027, #169, #17925 ) ;
#12610=EDGE_LOOP ( 'NONE', ( #21954, #19586, #24998, #18477 ) ) ;
#12640=ADVANCED_FACE ( 'NONE', ( #11487 ), #23034, .T. ) ;
#12642=DIRECTION ( 'NONE',  ( 0.8775825618903722036, 0.000000000000000000, -0.4794255386042041156 ) ) ;
#12647=ORIENTED_EDGE ( 'NONE', *, *, #23406, .T. ) ;
#12650=CARTESIAN_POINT ( 'NONE',  ( 27.18988201479999844, -20.30155444569999901, 49.77074518290000071 ) ) ;
#12652=CARTESIAN_POINT ( 'NONE',  ( -27.68682485439999752, -35.29999999999999716, -50.68039294919999804 ) ) ;
#12657=VERTEX_POINT ( 'NONE', #11638 ) ;
#12667=CARTESIAN_POINT ( 'NONE',  ( -9.348798002780000616, -10.50000000000000000, -17.11285995690000306 ) ) ;
#12670=DIRECTION ( 'NONE',  ( 0.000000000000000000, 1.000000000000000000, 0.000000000000000000 ) ) ;
#12671=CIRCLE ( 'NONE', #23857, 57.75000000000000000 ) ;
#12673=LINE ( 'NONE', #26386, #16707 ) ;
#12682=CIRCLE ( 'NONE', #15007, 0.4999999999999981126 ) ;
#12688=DIRECTION ( 'NONE',  ( 0.8775825618903722036, 0.000000000000000000, -0.4794255386042041156 ) ) ;
#12697=EDGE_CURVE ( 'NONE', #15179, #21477, #10430, .T. ) ;
#12700=LINE ( 'NONE', #15165, #24660 ) ;
#12704=EDGE_CURVE ( 'NONE', #19645, #12804, #21127, .T. ) ;
#12713=CARTESIAN_POINT ( 'NONE',  ( 0.000000000000000000, -39.50000000000000000, 0.000000000000000000 ) ) ;
#12714=AXIS2_PLACEMENT_3D ( 'NONE', #17330, #12790, #10588 ) ;
#12715=DIRECTION ( 'NONE',  ( 0.4794255386042033384, 0.000000000000000000, 0.8775825618903726477 ) ) ;
#12716=VECTOR ( 'NONE', #19611, 1000.000000000000000 ) ;
#12718=DIRECTION ( 'NONE',  ( 0.000000000000000000, -1.000000000000000000, 0.000000000000000000 ) ) ;
#12721=CARTESIAN_POINT ( 'NONE',  ( -31.00000000000000000, -11.00000000000000000, 4.500000000000000000 ) ) ;
#12725=CARTESIAN_POINT ( 'NONE',  ( -26.69293917519999937, -34.10310889129999623, -48.86109741659999628 ) ) ;
#12726=ORIENTED_EDGE ( 'NONE', *, *, #20297, .F. ) ;
#12734=DIRECTION ( 'NONE',  ( 0.4794255386042041156, 0.000000000000000000, 0.8775825618903720926 ) ) ;
#12751=CIRCLE ( 'NONE', #13240, 55.67692378859999991 ) ;
#12754=DIRECTION ( 'NONE',  ( 0.8775825618903722036, 0.000000000000000000, -0.4794255386042041156 ) ) ;
#12761=EDGE_CURVE ( 'NONE', #25949, #87, #8397, .T. ) ;
#12768=ORIENTED_EDGE ( 'NONE', *, *, #18470, .F. ) ;
#12773=EDGE_LOOP ( 'NONE', ( #17103, #1874, #21903, #24235 ) ) ;
#12790=DIRECTION ( 'NONE',  ( 0.000000000000000000, 1.000000000000000000, 0.000000000000000000 ) ) ;
#12798=DIRECTION ( 'NONE',  ( 0.000000000000000000, -1.000000000000000000, 0.000000000000000000 ) ) ;
#12804=VERTEX_POINT ( 'NONE', #13054 ) ;
#12812=CARTESIAN_POINT ( 'NONE',  ( -26.69293917519999937, -33.49689110869999809, -48.86109741659999628 ) ) ;
#12817=DIRECTION ( 'NONE',  ( 1.000000000000000000, 0.000000000000000000, 1.836909530729999990E-16 ) ) ;
#12823=VERTEX_POINT ( 'NONE', #21818 ) ;
#12831=ORIENTED_EDGE ( 'NONE', *, *, #24680, .F. ) ;
#12841=FACE_OUTER_BOUND ( 'NONE', #5444, .T. ) ;
#12843=EDGE_LOOP ( 'NONE', ( #16546, #21439, #23035, #28682 ) ) ;
#12847=ORIENTED_EDGE ( 'NONE', *, *, #7974, .F. ) ;
#12854=CARTESIAN_POINT ( 'NONE',  ( 4.500000000000000000, -15.00000000000000000, -31.00000000000000000 ) ) ;
#12863=EDGE_CURVE ( 'NONE', #27211, #5075, #7963, .T. ) ;
#12866=CARTESIAN_POINT ( 'NONE',  ( -27.68682485439999752, -20.89999999999999858, -50.68039294919999804 ) ) ;
#12876=EDGE_LOOP ( 'NONE', ( #6389, #11646, #15953, #18969 ) ) ;
#12877=LINE ( 'NONE', #6203, #19734 ) ;
#12890=ORIENTED_EDGE ( 'NONE', *, *, #18902, .T. ) ;
#12891=EDGE_CURVE ( 'NONE', #9393, #14188, #16854, .T. ) ;
#12893=CONICAL_SURFACE ( 'NONE', #2716, 57.74999999999999289, 1.224257462359999549 ) ;
#12895=ORIENTED_EDGE ( 'NONE', *, *, #10688, .F. ) ;
#12897=EDGE_CURVE ( 'NONE', #19426, #27931, #7365, .T. ) ;
#12905=ORIENTED_EDGE ( 'NONE', *, *, #10520, .F. ) ;
#12909=DIRECTION ( 'NONE',  ( 1.000000000000000000, 0.000000000000000000, 6.123031769109999188E-17 ) ) ;
#12935=DIRECTION ( 'NONE',  ( 0.4794255386042041156, 0.000000000000000000, 0.8775825618903722036 ) ) ;
#12939=FACE_OUTER_BOUND ( 'NONE', #13072, .T. ) ;
#12942=ORIENTED_EDGE ( 'NONE', *, *, #13339, .T. ) ;
#12945=VERTEX_POINT ( 'NONE', #14517 ) ;
#12956=ORIENTED_EDGE ( 'NONE', *, *, #15304, .T. ) ;
#12991=DIRECTION ( 'NONE',  ( 1.000000000000000000, 0.000000000000000000, 0.000000000000000000 ) ) ;
#12992=ORIENTED_EDGE ( 'NONE', *, *, #7024, .T. ) ;
#12998=ORIENTED_EDGE ( 'NONE', *, *, #17670, .F. ) ;
#13005=VERTEX_POINT ( 'NONE', #19594 ) ;
#13011=CARTESIAN_POINT ( 'NONE',  ( 0.000000000000000000, -37.57799544290000426, 0.000000000000000000 ) ) ;
#13015=ADVANCED_FACE ( 'NONE', ( #13173 ), #13864, .T. ) ;
#13025=ORIENTED_EDGE ( 'NONE', *, *, #4275, .F. ) ;
#13028=ORIENTED_EDGE ( 'NONE', *, *, #5573, .F. ) ;
#13037=CIRCLE ( 'NONE', #6553, 0.3500000000000003664 ) ;
#13051=ORIENTED_EDGE ( 'NONE', *, *, #2625, .T. ) ;
#13054=CARTESIAN_POINT ( 'NONE',  ( -4.500000000000000000, -15.00000000000000000, -31.00000000000000000 ) ) ;
#13058=DIRECTION ( 'NONE',  ( 1.000000000000000000, 0.000000000000000000, 0.000000000000000000 ) ) ;
#13062=CARTESIAN_POINT ( 'NONE',  ( 0.000000000000000000, -15.00000000000000000, 0.000000000000000000 ) ) ;
#13072=EDGE_LOOP ( 'NONE', ( #5365, #10655, #15349, #19298 ) ) ;
#13078=DIRECTION ( 'NONE',  ( 0.3422283636740854340, -0.7003189540771749266, 0.6264448177271558782 ) ) ;
#13085=CARTESIAN_POINT ( 'NONE',  ( -29.08514934200000113, -10.00000000000000000, -53.24000875469999983 ) ) ;
#13096=CARTESIAN_POINT ( 'NONE',  ( 0.000000000000000000, -34.10310889129999623, 0.000000000000000000 ) ) ;
#13100=ADVANCED_FACE ( 'NONE', ( #20780 ), #4553, .T. ) ;
#13101=CARTESIAN_POINT ( 'NONE',  ( 0.000000000000000000, -13.50000000000000000, 14.25000000000000000 ) ) ;
#13127=ORIENTED_EDGE ( 'NONE', *, *, #17200, .F. ) ;
#13128=CARTESIAN_POINT ( 'NONE',  ( -50.00000000000000000, -15.00000000000000000, -4.500000000000000000 ) ) ;
#13148=AXIS2_PLACEMENT_3D ( 'NONE', #15136, #1769, #19254 ) ;
#13156=CARTESIAN_POINT ( 'NONE',  ( -26.77683864449999973, -23.00000000000000000, -49.01467436490000296 ) ) ;
#13160=CONICAL_SURFACE ( 'NONE', #24342, 55.67692378859999280, 1.047197551199999799 ) ;
#13173=FACE_OUTER_BOUND ( 'NONE', #7019, .T. ) ;
#13175=EDGE_CURVE ( 'NONE', #18448, #17829, #22526, .T. ) ;
#13176=EDGE_CURVE ( 'NONE', #19773, #15453, #900, .T. ) ;
#13201=CIRCLE ( 'NONE', #9949, 9.500000000000001776 ) ;
#13202=DIRECTION ( 'NONE',  ( 1.000000000000000000, 0.000000000000000000, 0.000000000000000000 ) ) ;
#13216=ORIENTED_EDGE ( 'NONE', *, *, #2625, .F. ) ;
#13222=FACE_OUTER_BOUND ( 'NONE', #9317, .T. ) ;
#13227=CARTESIAN_POINT ( 'NONE',  ( 0.000000000000000000, -23.00000000000000000, 0.000000000000000000 ) ) ;
#13232=EDGE_CURVE ( 'NONE', #26990, #12325, #8851, .T. ) ;
#13233=AXIS2_PLACEMENT_3D ( 'NONE', #22631, #25109, #2671 ) ;
#13234=DIRECTION ( 'NONE',  ( 0.000000000000000000, -1.000000000000000000, 0.000000000000000000 ) ) ;
#13240=AXIS2_PLACEMENT_3D ( 'NONE', #3680, #18862, #17077 ) ;
#13241=ADVANCED_FACE ( 'NONE', ( #6541 ), #22736, .F. ) ;
#13262=ORIENTED_EDGE ( 'NONE', *, *, #9903, .T. ) ;
#13298=ORIENTED_EDGE ( 'NONE', *, *, #5286, .F. ) ;
#13312=EDGE_CURVE ( 'NONE', #13903, #640, #21791, .T. ) ;
#13327=CARTESIAN_POINT ( 'NONE',  ( 4.500000000000000000, -12.50000000000000000, 40.50000000000000000 ) ) ;
#13339=EDGE_CURVE ( 'NONE', #12657, #1944, #24763, .T. ) ;
#13346=DIRECTION ( 'NONE',  ( 0.000000000000000000, 1.000000000000000000, 0.000000000000000000 ) ) ;
#13348=DIRECTION ( 'NONE',  ( 0.000000000000000000, 1.000000000000000000, 0.000000000000000000 ) ) ;
#13352=CARTESIAN_POINT ( 'NONE',  ( 0.000000000000000000, -6.000000000000000000, 0.000000000000000000 ) ) ;
#13354=FACE_OUTER_BOUND ( 'NONE', #10697, .T. ) ;
#13361=EDGE_CURVE ( 'NONE', #11126, #258, #23652, .T. ) ;
#13365=VERTEX_POINT ( 'NONE', #22581 ) ;
#13375=ORIENTED_EDGE ( 'NONE', *, *, #12420, .F. ) ;
#13376=DIRECTION ( 'NONE',  ( 0.000000000000000000, 1.000000000000000000, 0.000000000000000000 ) ) ;
#13386=DIRECTION ( 'NONE',  ( -0.8775825618903722036, 0.000000000000000000, 0.4794255386042041156 ) ) ;
#13393=VERTEX_POINT ( 'NONE', #18199 ) ;
#13412=FACE_OUTER_BOUND ( 'NONE', #18168, .T. ) ;
#13425=CIRCLE ( 'NONE', #23235, 55.67692378859999991 ) ;
#13430=ORIENTED_EDGE ( 'NONE', *, *, #15898, .F. ) ;
#13441=DIRECTION ( 'NONE',  ( 1.000000000000000000, 0.000000000000000000, 0.000000000000000000 ) ) ;
#13456=CARTESIAN_POINT ( 'NONE',  ( 0.000000000000000000, -39.32601556110000018, 0.000000000000000000 ) ) ;
#13477=CARTESIAN_POINT ( 'NONE',  ( -6.831813925109999630, -11.50000000000000000, -12.50555150689999984 ) ) ;
#13479=DIRECTION ( 'NONE',  ( 1.000000000000000000, 0.000000000000000000, 0.000000000000000000 ) ) ;
#13494=DIRECTION ( 'NONE',  ( -0.8775825618903722036, 0.000000000000000000, 0.4794255386042041156 ) ) ;
#13499=EDGE_LOOP ( 'NONE', ( #24340, #14890, #23267, #12510 ) ) ;
#13500=ORIENTED_EDGE ( 'NONE', *, *, #18904, .T. ) ;
#13504=EDGE_LOOP ( 'NONE', ( #26782, #9710, #17916, #24371 ) ) ;
#13517=EDGE_CURVE ( 'NONE', #18513, #11029, #11534, .T. ) ;
#13520=DIRECTION ( 'NONE',  ( 0.4794255386042000078, 0.000000000000000000, 0.8775825618903743131 ) ) ;
#13527=CARTESIAN_POINT ( 'NONE',  ( 0.000000000000000000, -33.79999999999999716, 0.000000000000000000 ) ) ;
#13529=DIRECTION ( 'NONE',  ( 0.4794255386042040046, 0.000000000000000000, 0.8775825618903722036 ) ) ;
#13533=AXIS2_PLACEMENT_3D ( 'NONE', #26081, #25942, #14719 ) ;
#13538=CIRCLE ( 'NONE', #21020, 55.67692378859999991 ) ;
#13558=AXIS2_PLACEMENT_3D ( 'NONE', #17629, #13386, #12075 ) ;
#13561=EDGE_LOOP ( 'NONE', ( #9803, #14938, #8952, #8483 ) ) ;
#13571=AXIS2_PLACEMENT_3D ( 'NONE', #1704, #25887, #16575 ) ;
#13575=AXIS2_PLACEMENT_3D ( 'NONE', #15313, #2100, #25989 ) ;
#13589=DIRECTION ( 'NONE',  ( 0.000000000000000000, 1.000000000000000000, 0.000000000000000000 ) ) ;
#13592=ORIENTED_EDGE ( 'NONE', *, *, #17008, .T. ) ;
#13611=ORIENTED_EDGE ( 'NONE', *, *, #1381, .T. ) ;
#13630=CARTESIAN_POINT ( 'NONE',  ( 12.03978574509999966, -15.50000000000000000, 22.03867997850000293 ) ) ;
#13631=VECTOR ( 'NONE', #5560, 1000.000000000000000 ) ;
#13633=DIRECTION ( 'NONE',  ( -0.000000000000000000, 1.000000000000000000, 0.000000000000000000 ) ) ;
#13634=CARTESIAN_POINT ( 'NONE',  ( -40.50000000000000000, -11.00000000000000000, -4.500000000000000000 ) ) ;
#13643=DIRECTION ( 'NONE',  ( 0.000000000000000000, 1.000000000000000000, 0.000000000000000000 ) ) ;
#13645=ORIENTED_EDGE ( 'NONE', *, *, #23898, .F. ) ;
#13652=EDGE_CURVE ( 'NONE', #14525, #17829, #1337, .T. ) ;
#13655=EDGE_CURVE ( 'NONE', #8384, #3189, #21328, .T. ) ;
#13670=ORIENTED_EDGE ( 'NONE', *, *, #5733, .F. ) ;
#13675=CARTESIAN_POINT ( 'NONE',  ( 0.000000000000000000, -28.10000000000000142, 0.000000000000000000 ) ) ;
#13676=DIRECTION ( 'NONE',  ( 1.000000000000000000, 0.000000000000000000, 0.000000000000000000 ) ) ;
#13681=DIRECTION ( 'NONE',  ( 0.4151946956541399669, 0.5000000000001689759, 0.7600087925152558821 ) ) ;
#13688=VECTOR ( 'NONE', #23125, 999.9999999999998863 ) ;
#13699=AXIS2_PLACEMENT_3D ( 'NONE', #9252, #25000, #4599 ) ;
#13708=LINE ( 'NONE', #9477, #24634 ) ;
#13716=CARTESIAN_POINT ( 'NONE',  ( 0.000000000000000000, -36.20000000000000284, 0.000000000000000000 ) ) ;
#13735=ORIENTED_EDGE ( 'NONE', *, *, #15543, .T. ) ;
#13746=ADVANCED_FACE ( 'NONE', ( #10549 ), #18577, .F. ) ;
#13760=LINE ( 'NONE', #15789, #24146 ) ;
#13769=ORIENTED_EDGE ( 'NONE', *, *, #27863, .T. ) ;
#13774=ORIENTED_EDGE ( 'NONE', *, *, #17596, .F. ) ;
#13778=DIRECTION ( 'NONE',  ( 1.000000000000000000, 0.000000000000000000, 0.000000000000000000 ) ) ;
#13793=CARTESIAN_POINT ( 'NONE',  ( 28.07036528529999941, -39.50000000000000000, 51.38245899869999533 ) ) ;
#13795=AXIS2_PLACEMENT_3D ( 'NONE', #7627, #6252, #12513 ) ;
#13811=FACE_OUTER_BOUND ( 'NONE', #8984, .T. ) ;
#13837=CARTESIAN_POINT ( 'NONE',  ( 0.000000000000000000, -2.000000000000000000, 0.000000000000000000 ) ) ;
#13838=AXIS2_PLACEMENT_3D ( 'NONE', #22130, #20371, #9140 ) ;
#13841=ORIENTED_EDGE ( 'NONE', *, *, #5286, .T. ) ;
#13847=CONICAL_SURFACE ( 'NONE', #2696, 55.67692378859999280, 1.047197551199999799 ) ;
#13864=TOROIDAL_SURFACE ( 'NONE', #12001, 24.50000000000000000, 3.000000000000000000 ) ;
#13872=CARTESIAN_POINT ( 'NONE',  ( 26.77683864449999973, -26.59999999999999787, 49.01467436490000296 ) ) ;
#13882=AXIS2_PLACEMENT_3D ( 'NONE', #4644, #11329, #13520 ) ;
#13891=CARTESIAN_POINT ( 'NONE',  ( -28.31007805460000171, -40.00000000000000000, -51.82125027960000097 ) ) ;
#13898=DIRECTION ( 'NONE',  ( 0.000000000000000000, 1.000000000000000000, 0.000000000000000000 ) ) ;
#13903=VERTEX_POINT ( 'NONE', #11135 ) ;
#13919=AXIS2_PLACEMENT_3D ( 'NONE', #15386, #11316, #17895 ) ;
#13926=EDGE_CURVE ( 'NONE', #4628, #6607, #6353, .T. ) ;
#13940=ORIENTED_EDGE ( 'NONE', *, *, #23610, .T. ) ;
#13941=CIRCLE ( 'NONE', #25576, 21.60095686220000033 ) ;
#13977=ORIENTED_EDGE ( 'NONE', *, *, #28515, .T. ) ;
#13987=VERTEX_POINT ( 'NONE', #10698 ) ;
#13988=AXIS2_PLACEMENT_3D ( 'NONE', #6812, #13494, #22402 ) ;
#13992=DIRECTION ( 'NONE',  ( 0.8775825618903722036, 0.000000000000000000, -0.4794255386042041156 ) ) ;
#13998=DIRECTION ( 'NONE',  ( 0.4151946956541399669, 0.5000000000001689759, 0.7600087925152558821 ) ) ;
#14004=DIRECTION ( 'NONE',  ( 0.4707989697561778542, 0.1888473936500709438, 0.8617917335343248109 ) ) ;
#14005=CARTESIAN_POINT ( 'NONE',  ( 26.69293917519999937, -26.90310889129999694, 48.86109741659999628 ) ) ;
#14009=FACE_OUTER_BOUND ( 'NONE', #21262, .T. ) ;
#14011=VERTEX_POINT ( 'NONE', #28639 ) ;
#14025=AXIS2_PLACEMENT_3D ( 'NONE', #18750, #12307, #21216 ) ;
#14035=FACE_OUTER_BOUND ( 'NONE', #20062, .T. ) ;
#14046=LINE ( 'NONE', #3137, #9047 ) ;
#14052=EDGE_LOOP ( 'NONE', ( #14329, #5984, #15787, #22212 ) ) ;
#14062=CARTESIAN_POINT ( 'NONE',  ( 0.000000000000000000, -19.70310889130000120, 0.000000000000000000 ) ) ;
#14064=EDGE_CURVE ( 'NONE', #19645, #12096, #23671, .T. ) ;
#14066=SURFACE_STYLE_FILL_AREA ( #20923 ) ;
#14070=EDGE_LOOP ( 'NONE', ( #21576, #18820, #21323, #18973 ) ) ;
#14086=CARTESIAN_POINT ( 'NONE',  ( -27.18988201479999844, -16.70155444569999759, -49.77074518290000071 ) ) ;
#14093=ADVANCED_FACE ( 'NONE', ( #22547 ), #5200, .T. ) ;
#14100=ORIENTED_EDGE ( 'NONE', *, *, #8390, .T. ) ;
#14118=ADVANCED_FACE ( 'NONE', ( #999 ), #454, .T. ) ;
#14140=ORIENTED_EDGE ( 'NONE', *, *, #1947, .T. ) ;
#14160=CIRCLE ( 'NONE', #16960, 55.67692378859999991 ) ;
#14169=EDGE_CURVE ( 'NONE', #26731, #1871, #16225, .T. ) ;
#14176=ORIENTED_EDGE ( 'NONE', *, *, #2528, .T. ) ;
#14188=VERTEX_POINT ( 'NONE', #12721 ) ;
#14197=DIRECTION ( 'NONE',  ( 0.000000000000000000, 1.000000000000000000, 0.000000000000000000 ) ) ;
#14199=DIRECTION ( 'NONE',  ( -1.000000000000000000, 0.000000000000000000, -1.836909530729999990E-16 ) ) ;
#14205=CARTESIAN_POINT ( 'NONE',  ( 27.18988201479999844, -18.49844555430000170, 49.77074518290000071 ) ) ;
#14206=CARTESIAN_POINT ( 'NONE',  ( 0.000000000000000000, -30.50310889129999836, 0.000000000000000000 ) ) ;
#14220=FILL_AREA_STYLE_COLOUR ( '', #18293 ) ;
#14229=CARTESIAN_POINT ( 'NONE',  ( 29.17304402409999753, -39.50000000000000000, 53.40089889099999709 ) ) ;
#14272=VERTEX_POINT ( 'NONE', #19581 ) ;
#14280=VERTEX_POINT ( 'NONE', #26154 ) ;
#14290=DIRECTION ( 'NONE',  ( 0.8775825618903722036, 0.000000000000000000, -0.4794255386042041156 ) ) ;
#14292=ORIENTED_EDGE ( 'NONE', *, *, #22620, .F. ) ;
#14304=DIRECTION ( 'NONE',  ( 0.4794255386042040046, 0.000000000000000000, 0.8775825618903722036 ) ) ;
#14309=ADVANCED_FACE ( 'NONE', ( #20165 ), #21347, .T. ) ;
#14314=DIRECTION ( 'NONE',  ( -0.000000000000000000, 1.000000000000000000, 0.000000000000000000 ) ) ;
#14320=CYLINDRICAL_SURFACE ( 'NONE', #2023, 9.500000000000001776 ) ;
#14323=ORIENTED_EDGE ( 'NONE', *, *, #3278, .T. ) ;
#14329=ORIENTED_EDGE ( 'NONE', *, *, #7024, .F. ) ;
#14332=DIRECTION ( 'NONE',  ( 0.000000000000000000, 1.000000000000000000, 0.000000000000000000 ) ) ;
#14333=DIRECTION ( 'NONE',  ( 0.000000000000000000, 1.000000000000000000, 0.000000000000000000 ) ) ;
#14344=AXIS2_PLACEMENT_3D ( 'NONE', #3700, #18735, #21200 ) ;
#14348=DIRECTION ( 'NONE',  ( 0.000000000000000000, 1.000000000000000000, 0.000000000000000000 ) ) ;
#14358=ORIENTED_EDGE ( 'NONE', *, *, #11016, .F. ) ;
#14359=ADVANCED_FACE ( 'NONE', ( #22357 ), #6465, .T. ) ;
#14368=AXIS2_PLACEMENT_3D ( 'NONE', #3337, #16003, #18790 ) ;
#14372=CARTESIAN_POINT ( 'NONE',  ( 0.000000000000000000, -33.79999999999999716, 0.000000000000000000 ) ) ;
#14385=AXIS2_PLACEMENT_3D ( 'NONE', #10761, #8878, #31 ) ;
#14393=DIRECTION ( 'NONE',  ( 0.000000000000000000, 1.000000000000000000, 0.000000000000000000 ) ) ;
#14401=VERTEX_POINT ( 'NONE', #21920 ) ;
#14402=CIRCLE ( 'NONE', #11592, 55.50192378860000275 ) ;
#14405=DIRECTION ( 'NONE',  ( 1.000000000000000000, 0.000000000000000000, 0.000000000000000000 ) ) ;
#14415=CARTESIAN_POINT ( 'NONE',  ( 2.220446049249999745E-14, -15.00000000000000000, -31.00000000000000000 ) ) ;
#14417=EDGE_CURVE ( 'NONE', #5336, #11019, #10638, .T. ) ;
#14422=ORIENTED_EDGE ( 'NONE', *, *, #12389, .F. ) ;
#14423=DIRECTION ( 'NONE',  ( 1.000000000000000000, 0.000000000000000000, 0.000000000000000000 ) ) ;
#14424=TOROIDAL_SURFACE ( 'NONE', #12540, 52.35000000000000142, 1.000000000000000000 ) ;
#14426=VERTEX_POINT ( 'NONE', #21447 ) ;
#14432=DIRECTION ( 'NONE',  ( 0.000000000000000000, 0.000000000000000000, -1.000000000000000000 ) ) ;
#14434=CARTESIAN_POINT ( 'NONE',  ( 0.000000000000000000, -17.50000000000000000, 0.000000000000000000 ) ) ;
#14446=AXIS2_PLACEMENT_3D ( 'NONE', #6946, #3574, #5614 ) ;
#14447=SHAPE_REPRESENTATION_RELATIONSHIP ( 'NONE' , 'NONE' ,  #5912, #25525 ) ;
#14458=CARTESIAN_POINT ( 'NONE',  ( 0.000000000000000000, -21.50000000000000000, 0.000000000000000000 ) ) ;
#14459=EDGE_CURVE ( 'NONE', #9863, #77, #7435, .T. ) ;
#14465=VECTOR ( 'NONE', #15295, 1000.000000000000000 ) ;
#14485=CARTESIAN_POINT ( 'NONE',  ( -26.60903970598167589, -19.40000000000000213, -48.70752046822583736 ) ) ;
#14488=ORIENTED_EDGE ( 'NONE', *, *, #7673, .F. ) ;
#14500=VECTOR ( 'NONE', #18446, 1000.000000000000000 ) ;
#14502=EDGE_CURVE ( 'NONE', #87, #3592, #22300, .T. ) ;
#14503=DIRECTION ( 'NONE',  ( 0.000000000000000000, 0.000000000000000000, 1.000000000000000000 ) ) ;
#14505=FACE_OUTER_BOUND ( 'NONE', #9039, .T. ) ;
#14516=VECTOR ( 'NONE', #7177, 1000.000000000000114 ) ;
#14517=CARTESIAN_POINT ( 'NONE',  ( 26.60903970598167589, -19.40000000000000213, 48.70752046822583736 ) ) ;
#14520=LINE ( 'NONE', #18775, #6186 ) ;
#14525=VERTEX_POINT ( 'NONE', #20119 ) ;
#14532=AXIS2_PLACEMENT_3D ( 'NONE', #22485, #20437, #22332 ) ;
#14542=ADVANCED_FACE ( 'NONE', ( #2355 ), #1383, .F. ) ;
#14543=EDGE_CURVE ( 'NONE', #8365, #23467, #21833, .T. ) ;
#14561=ORIENTED_EDGE ( 'NONE', *, *, #17105, .F. ) ;
#14572=EDGE_CURVE ( 'NONE', #2880, #11154, #22776, .T. ) ;
#14574=DIRECTION ( 'NONE',  ( 0.4794255386042036160, 0.000000000000000000, 0.8775825618903723147 ) ) ;
#14575=CARTESIAN_POINT ( 'NONE',  ( 0.000000000000000000, -6.000000000000000000, 0.000000000000000000 ) ) ;
#14605=CARTESIAN_POINT ( 'NONE',  ( -3.883346862689999845, -9.250000000000000000, -7.108418751309999450 ) ) ;
#14620=CARTESIAN_POINT ( 'NONE',  ( -27.68682485439999752, -24.80000000000000071, -50.68039294919999804 ) ) ;
#14628=EDGE_CURVE ( 'NONE', #26186, #26809, #5123, .T. ) ;
#14630=DIRECTION ( 'NONE',  ( 0.000000000000000000, 1.000000000000000000, 0.000000000000000000 ) ) ;
#14649=ORIENTED_EDGE ( 'NONE', *, *, #3278, .F. ) ;
#14673=ORIENTED_EDGE ( 'NONE', *, *, #27291, .F. ) ;
#14675=LINE ( 'NONE', #22765, #19490 ) ;
#14678=ORIENTED_EDGE ( 'NONE', *, *, #22245, .T. ) ;
#14683=EDGE_LOOP ( 'NONE', ( #27152, #4586, #2026, #22031 ) ) ;
#14718=( NAMED_UNIT ( * ) SI_UNIT ( $, .STERADIAN. ) SOLID_ANGLE_UNIT ( ) );
#14719=DIRECTION ( 'NONE',  ( 0.4794255386042000078, 0.000000000000000000, 0.8775825618903743131 ) ) ;
#14721=DIRECTION ( 'NONE',  ( -0.8775825618903722036, 0.000000000000000000, 0.4794255386042041156 ) ) ;
#14732=ADVANCED_FACE ( 'NONE', ( #20231 ), #24603, .T. ) ;
#14739=DIRECTION ( 'NONE',  ( 0.4151946956541399669, 0.5000000000001689759, 0.7600087925152558821 ) ) ;
#14759=DIRECTION ( 'NONE',  ( 1.000000000000000000, 0.000000000000000000, 0.000000000000000000 ) ) ;
#14769=AXIS2_PLACEMENT_3D ( 'NONE', #20461, #7357, #4874 ) ;
#14776=FACE_BOUND ( 'NONE', #9834, .T. ) ;
#14777=EDGE_LOOP ( 'NONE', ( #23806, #21338, #8046, #12905 ) ) ;
#14800=CARTESIAN_POINT ( 'NONE',  ( 50.00000000000000000, 0.000000000000000000, -4.500000000000000000 ) ) ;
#14804=DIRECTION ( 'NONE',  ( 0.000000000000000000, 1.000000000000000000, 0.000000000000000000 ) ) ;
#14816=CARTESIAN_POINT ( 'NONE',  ( -28.54979082390000045, -12.59999999999999964, -52.26004156059999417 ) ) ;
#14817=ORIENTED_EDGE ( 'NONE', *, *, #26826, .F. ) ;
#14841=ORIENTED_EDGE ( 'NONE', *, *, #20330, .T. ) ;
#14845=DIRECTION ( 'NONE',  ( 0.000000000000000000, -1.000000000000000000, 0.000000000000000000 ) ) ;
#14869=AXIS2_PLACEMENT_3D ( 'NONE', #4765, #4321, #20055 ) ;
#14875=AXIS2_PLACEMENT_3D ( 'NONE', #7231, #6642, #8950 ) ;
#14890=ORIENTED_EDGE ( 'NONE', *, *, #18238, .T. ) ;
#14898=DIRECTION ( 'NONE',  ( 1.000000000000000000, 0.000000000000000000, 0.000000000000000000 ) ) ;
#14902=CARTESIAN_POINT ( 'NONE',  ( 29.17304402409999753, -10.50000000000000000, 53.40089889099999709 ) ) ;
#14906=CARTESIAN_POINT ( 'NONE',  ( 27.18988201479999844, -27.50155444569999830, 49.77074518290000071 ) ) ;
#14911=AXIS2_PLACEMENT_3D ( 'NONE', #17360, #21451, #17506 ) ;
#14912=ORIENTED_EDGE ( 'NONE', *, *, #11591, .F. ) ;
#14918=AXIS2_PLACEMENT_3D ( 'NONE', #10839, #4161, #8811 ) ;
#14920=ADVANCED_FACE ( 'NONE', ( #25043 ), #12054, .F. ) ;
#14938=ORIENTED_EDGE ( 'NONE', *, *, #8030, .T. ) ;
#14976=EDGE_LOOP ( 'NONE', ( #11218, #1988, #21396, #13645 ) ) ;
#14995=AXIS2_PLACEMENT_3D ( 'NONE', #22322, #8471, #24066 ) ;
#14999=EDGE_LOOP ( 'NONE', ( #2058, #7769, #8903, #9297 ) ) ;
#15003=CARTESIAN_POINT ( 'NONE',  ( -50.00000000000000000, 0.000000000000000000, 4.500000000000000000 ) ) ;
#15007=AXIS2_PLACEMENT_3D ( 'NONE', #16933, #25538, #20893 ) ;
#15017=CARTESIAN_POINT ( 'NONE',  ( 0.000000000000000000, -37.57799544290000426, 0.000000000000000000 ) ) ;
#15021=AXIS2_PLACEMENT_3D ( 'NONE', #9400, #18154, #13778 ) ;
#15022=CARTESIAN_POINT ( 'NONE',  ( -28.44874375979999925, -10.08849557519999962, -52.07507615039999394 ) ) ;
#15025=DIRECTION ( 'NONE',  ( -0.3390050494208429743, 0.7071067811866730279, -0.6205445805637129775 ) ) ;
#15029=CARTESIAN_POINT ( 'NONE',  ( 27.68682485439999752, -24.80000000000000071, 50.68039294919999804 ) ) ;
#15035=ORIENTED_EDGE ( 'NONE', *, *, #15531, .F. ) ;
#15042=DIRECTION ( 'NONE',  ( 0.000000000000000000, 1.000000000000000000, 0.000000000000000000 ) ) ;
#15064=ORIENTED_EDGE ( 'NONE', *, *, #3244, .F. ) ;
#15085=ORIENTED_EDGE ( 'NONE', *, *, #11467, .T. ) ;
#15100=ADVANCED_FACE ( 'NONE', ( #5005 ), #231, .F. ) ;
#15101=DIRECTION ( 'NONE',  ( 0.4794255386042059475, 0.000000000000000000, 0.8775825618903710934 ) ) ;
#15124=CARTESIAN_POINT ( 'NONE',  ( 4.500000000000000000, 0.000000000000000000, -31.00000000000000000 ) ) ;
#15136=CARTESIAN_POINT ( 'NONE',  ( 0.000000000000000000, -16.00000000000000000, 0.000000000000000000 ) ) ;
#15138=CIRCLE ( 'NONE', #4950, 8.099999999999999645 ) ;
#15157=ORIENTED_EDGE ( 'NONE', *, *, #19056, .T. ) ;
#15165=CARTESIAN_POINT ( 'NONE',  ( 4.123059632000000363, -17.00000000000000000, 7.547210032260000645 ) ) ;
#15175=DIRECTION ( 'NONE',  ( 0.4794255386042041156, 0.000000000000000000, 0.8775825618903720926 ) ) ;
#15179=VERTEX_POINT ( 'NONE', #18715 ) ;
#15183=CARTESIAN_POINT ( 'NONE',  ( 0.000000000000000000, -10.50000000000000000, 0.000000000000000000 ) ) ;
#15189=EDGE_CURVE ( 'NONE', #23053, #14525, #9805, .T. ) ;
#15191=EDGE_CURVE ( 'NONE', #20122, #5395, #1401, .T. ) ;
#15202=ORIENTED_EDGE ( 'NONE', *, *, #14064, .T. ) ;
#15215=ORIENTED_EDGE ( 'NONE', *, *, #16888, .T. ) ;
#15237=ORIENTED_EDGE ( 'NONE', *, *, #10481, .F. ) ;
#15238=FACE_OUTER_BOUND ( 'NONE', #17823, .T. ) ;
#15242=CARTESIAN_POINT ( 'NONE',  ( -11.69905354509999995, -15.49681045920000066, -21.41497386989999896 ) ) ;
#15252=ORIENTED_EDGE ( 'NONE', *, *, #19596, .F. ) ;
#15256=DIRECTION ( 'NONE',  ( 0.000000000000000000, 1.000000000000000000, 0.000000000000000000 ) ) ;
#15263=ADVANCED_FACE ( 'NONE', ( #7119 ), #11454, .F. ) ;
#15268=ORIENTED_EDGE ( 'NONE', *, *, #26160, .F. ) ;
#15280=EDGE_LOOP ( 'NONE', ( #28039, #16262, #22942, #18403 ) ) ;
#15286=DIRECTION ( 'NONE',  ( 0.3390050494208429743, 0.7071067811866730279, 0.6205445805637129775 ) ) ;
#15290=CARTESIAN_POINT ( 'NONE',  ( -26.77683864449999973, -19.40000000000000213, -49.01467436490000296 ) ) ;
#15295=DIRECTION ( 'NONE',  ( 0.000000000000000000, 1.000000000000000000, 0.000000000000000000 ) ) ;
#15304=EDGE_CURVE ( 'NONE', #1181, #914, #25133, .T. ) ;
#15305=ADVANCED_FACE ( 'NONE', ( #13354 ), #24184, .T. ) ;
#15313=CARTESIAN_POINT ( 'NONE',  ( 0.000000000000000000, -11.00000000000000000, 0.000000000000000000 ) ) ;
#15330=DIRECTION ( 'NONE',  ( 0.4794255386042040601, 0.000000000000000000, 0.8775825618903720926 ) ) ;
#15337=EDGE_LOOP ( 'NONE', ( #19855, #26371, #18389, #18841 ) ) ;
#15343=CIRCLE ( 'NONE', #27509, 57.73884739369999863 ) ;
#15349=ORIENTED_EDGE ( 'NONE', *, *, #25882, .F. ) ;
#15357=AXIS2_PLACEMENT_3D ( 'NONE', #15440, #22466, #22614 ) ;
#15358=FACE_BOUND ( 'NONE', #2339, .T. ) ;
#15361=VECTOR ( 'NONE', #1360, 1000.000000000000000 ) ;
#15363=CARTESIAN_POINT ( 'NONE',  ( -26.60903970598167589, -26.59999999999999787, -48.70752046822583736 ) ) ;
#15368=EDGE_CURVE ( 'NONE', #21532, #16418, #21851, .T. ) ;
#15386=CARTESIAN_POINT ( 'NONE',  ( -4.500000000000000000, -11.00000000000000000, -40.50000000000000000 ) ) ;
#15395=VERTEX_POINT ( 'NONE', #27790 ) ;
#15396=EDGE_CURVE ( 'NONE', #22021, #3254, #12453, .T. ) ;
#15402=DIRECTION ( 'NONE',  ( 0.000000000000000000, 1.000000000000000000, 0.000000000000000000 ) ) ;
#15407=ORIENTED_EDGE ( 'NONE', *, *, #3689, .T. ) ;
#15418=ORIENTED_EDGE ( 'NONE', *, *, #26851, .F. ) ;
#15431=CARTESIAN_POINT ( 'NONE',  ( 4.500000000000000000, -12.50000000000000000, -40.50000000000000000 ) ) ;
#15440=CARTESIAN_POINT ( 'NONE',  ( 0.000000000000000000, -26.29689110869999880, 0.000000000000000000 ) ) ;
#15441=EDGE_LOOP ( 'NONE', ( #22174, #12942, #26162, #11081 ) ) ;
#15452=CIRCLE ( 'NONE', #19194, 52.20000000000000284 ) ;
#15453=VERTEX_POINT ( 'NONE', #17129 ) ;
#15456=ORIENTED_EDGE ( 'NONE', *, *, #5933, .T. ) ;
#15462=DIRECTION ( 'NONE',  ( 1.000000000000000000, 0.000000000000000000, 0.000000000000000000 ) ) ;
#15466=CARTESIAN_POINT ( 'NONE',  ( -12.03978574509999966, -15.50000000000000000, -22.03867997850000293 ) ) ;
#15468=ORIENTED_EDGE ( 'NONE', *, *, #11016, .T. ) ;
#15472=EDGE_CURVE ( 'NONE', #914, #28370, #22817, .T. ) ;
#15477=ORIENTED_EDGE ( 'NONE', *, *, #13175, .F. ) ;
#15480=FACE_OUTER_BOUND ( 'NONE', #6183, .T. ) ;
#15488=FACE_OUTER_BOUND ( 'NONE', #10664, .T. ) ;
#15490=ORIENTED_EDGE ( 'NONE', *, *, #7161, .T. ) ;
#15502=VERTEX_POINT ( 'NONE', #17716 ) ;
#15504=DIRECTION ( 'NONE',  ( -0.8775825618903722036, 0.000000000000000000, 0.4794255386042041156 ) ) ;
#15509=CARTESIAN_POINT ( 'NONE',  ( 0.000000000000000000, -19.40000000000000213, 0.000000000000000000 ) ) ;
#15512=DIRECTION ( 'NONE',  ( 1.000000000000000000, 0.000000000000000000, 0.000000000000000000 ) ) ;
#15517=EDGE_LOOP ( 'NONE', ( #3501, #25677, #12998, #10536 ) ) ;
#15531=EDGE_CURVE ( 'NONE', #5075, #3752, #23731, .T. ) ;
#15538=CIRCLE ( 'NONE', #1618, 0.3500000000000003664 ) ;
#15543=EDGE_CURVE ( 'NONE', #18513, #22875, #18, .T. ) ;
#15544=ORIENTED_EDGE ( 'NONE', *, *, #6241, .T. ) ;
#15547=TOROIDAL_SURFACE ( 'NONE', #27681, 55.85192378860000417, 0.3499999999999999778 ) ;
#15550=DIRECTION ( 'NONE',  ( 0.4794255386042036715, 0.000000000000000000, 0.8775825618903724257 ) ) ;
#15555=CARTESIAN_POINT ( 'NONE',  ( 0.000000000000000000, -10.50000000000000000, 0.000000000000000000 ) ) ;
#15565=CARTESIAN_POINT ( 'NONE',  ( 27.68682485439999752, -20.89999999999999858, 50.68039294919999804 ) ) ;
#15566=CARTESIAN_POINT ( 'NONE',  ( 27.68682485439999752, -36.20000000000000284, 50.68039294919999804 ) ) ;
#15580=EDGE_CURVE ( 'NONE', #8526, #15179, #12421, .T. ) ;
#15588=DIRECTION ( 'NONE',  ( 0.4794255386042036715, 0.000000000000000000, 0.8775825618903723147 ) ) ;
#15594=LINE ( 'NONE', #15735, #27527 ) ;
#15620=VERTEX_POINT ( 'NONE', #22821 ) ;
#15639=ORIENTED_EDGE ( 'NONE', *, *, #21358, .F. ) ;
#15656=ORIENTED_EDGE ( 'NONE', *, *, #157, .T. ) ;
#15673=VERTEX_POINT ( 'NONE', #9682 ) ;
#15688=VERTEX_POINT ( 'NONE', #21070 ) ;
#15692=AXIS2_PLACEMENT_3D ( 'NONE', #4708, #11537, #26718 ) ;
#15694=DIRECTION ( 'NONE',  ( 0.000000000000000000, -1.000000000000000000, 0.000000000000000000 ) ) ;
#15695=CARTESIAN_POINT ( 'NONE',  ( -26.69293917519999937, -16.10310889129999623, -48.86109741659999628 ) ) ;
#15711=CARTESIAN_POINT ( 'NONE',  ( -50.00000000000000000, -15.00000000000000000, 4.500000000000000000 ) ) ;
#15712=CARTESIAN_POINT ( 'NONE',  ( 0.000000000000000000, -19.09689110869999951, 0.000000000000000000 ) ) ;
#15720=DIRECTION ( 'NONE',  ( 1.000000000000000000, 0.000000000000000000, 0.000000000000000000 ) ) ;
#15733=AXIS2_PLACEMENT_3D ( 'NONE', #2858, #6932, #11275 ) ;
#15734=DIRECTION ( 'NONE',  ( 0.000000000000000000, 1.000000000000000000, 0.000000000000000000 ) ) ;
#15735=CARTESIAN_POINT ( 'NONE',  ( -26.72663706610000034, -37.96100227850000408, -48.92278099219999632 ) ) ;
#15740=DIRECTION ( 'NONE',  ( 0.4794255386042036715, 0.000000000000000000, 0.8775825618903724257 ) ) ;
#15743=EDGE_CURVE ( 'NONE', #15688, #3752, #19567, .T. ) ;
#15751=DIRECTION ( 'NONE',  ( 1.000000000000000000, 0.000000000000000000, 0.000000000000000000 ) ) ;
#15754=AXIS2_PLACEMENT_3D ( 'NONE', #15993, #15845, #12165 ) ;
#15761=ORIENTED_EDGE ( 'NONE', *, *, #18871, .F. ) ;
#15777=FACE_OUTER_BOUND ( 'NONE', #11847, .T. ) ;
#15781=AXIS2_PLACEMENT_3D ( 'NONE', #13327, #26608, #20334 ) ;
#15787=ORIENTED_EDGE ( 'NONE', *, *, #27291, .T. ) ;
#15789=CARTESIAN_POINT ( 'NONE',  ( -1.865174681369999824E-14, -11.00000000000000000, 31.00000000000000000 ) ) ;
#15796=CIRCLE ( 'NONE', #21850, 55.67692378859999991 ) ;
#15810=DIRECTION ( 'NONE',  ( 0.000000000000000000, -1.000000000000000000, 0.000000000000000000 ) ) ;
#15823=ORIENTED_EDGE ( 'NONE', *, *, #13339, .F. ) ;
#15828=CYLINDRICAL_SURFACE ( 'NONE', #16963, 61.34999999999998721 ) ;
#15839=TOROIDAL_SURFACE ( 'NONE', #6529, 53.85000000000000142, 0.5000000000000000000 ) ;
#15842=AXIS2_PLACEMENT_3D ( 'NONE', #25116, #9063, #16360 ) ;
#15845=DIRECTION ( 'NONE',  ( 0.000000000000000000, 1.000000000000000000, 0.000000000000000000 ) ) ;
#15848=CARTESIAN_POINT ( 'NONE',  ( 0.000000000000000000, -2.000000000000000000, 0.000000000000000000 ) ) ;
#15851=DIRECTION ( 'NONE',  ( 0.000000000000000000, 1.000000000000000000, 0.000000000000000000 ) ) ;
#15853=FACE_OUTER_BOUND ( 'NONE', #26086, .T. ) ;
#15854=DIRECTION ( 'NONE',  ( 0.000000000000000000, 1.000000000000000000, 0.000000000000000000 ) ) ;
#15862=DIRECTION ( 'NONE',  ( 0.000000000000000000, 1.000000000000000000, 0.000000000000000000 ) ) ;
#15866=CIRCLE ( 'NONE', #13533, 0.3500000000000003664 ) ;
#15875=ORIENTED_EDGE ( 'NONE', *, *, #12125, .T. ) ;
#15888=DIRECTION ( 'NONE',  ( 1.000000000000000000, 0.000000000000000000, 0.000000000000000000 ) ) ;
#15898=EDGE_CURVE ( 'NONE', #4998, #22563, #859, .T. ) ;
#15911=ORIENTED_EDGE ( 'NONE', *, *, #15368, .T. ) ;
#15919=DIRECTION ( 'NONE',  ( -0.4751828347227322613, 0.1327433628319252545, -0.8698163445285104212 ) ) ;
#15934=ORIENTED_EDGE ( 'NONE', *, *, #10541, .F. ) ;
#15938=CARTESIAN_POINT ( 'NONE',  ( 0.000000000000000000, -32.30000000000000426, 0.000000000000000000 ) ) ;
#15947=EDGE_CURVE ( 'NONE', #11019, #5336, #369, .T. ) ;
#15953=ORIENTED_EDGE ( 'NONE', *, *, #14628, .T. ) ;
#15981=DIRECTION ( 'NONE',  ( 0.000000000000000000, 1.000000000000000000, 0.000000000000000000 ) ) ;
#15982=ORIENTED_EDGE ( 'NONE', *, *, #21876, .T. ) ;
#15987=CONICAL_SURFACE ( 'NONE', #20194, 57.74999999999999289, 1.224257462359999549 ) ;
#15988=DIRECTION ( 'NONE',  ( 0.000000000000000000, -1.000000000000000000, 0.000000000000000000 ) ) ;
#15993=CARTESIAN_POINT ( 'NONE',  ( 0.000000000000000000, -26.59999999999999787, 0.000000000000000000 ) ) ;
#16003=DIRECTION ( 'NONE',  ( 0.000000000000000000, 1.000000000000000000, 0.000000000000000000 ) ) ;
#16011=FACE_OUTER_BOUND ( 'NONE', #9629, .T. ) ;
#16013=DIRECTION ( 'NONE',  ( 1.000000000000000000, 0.000000000000000000, 0.000000000000000000 ) ) ;
#16020=ORIENTED_EDGE ( 'NONE', *, *, #8123, .F. ) ;
#16024=CIRCLE ( 'NONE', #24407, 0.3500000000000003664 ) ;
#16026=VERTEX_POINT ( 'NONE', #16509 ) ;
#16043=ORIENTED_EDGE ( 'NONE', *, *, #8427, .F. ) ;
#16046=AXIS2_PLACEMENT_3D ( 'NONE', #11405, #13898, #25285 ) ;
#16049=LINE ( 'NONE', #24951, #577 ) ;
#16056=TOROIDAL_SURFACE ( 'NONE', #13233, 60.85000000000000142, 0.5000000000000000000 ) ;
#16058=ORIENTED_EDGE ( 'NONE', *, *, #5318, .T. ) ;
#16065=LINE ( 'NONE', #11247, #26464 ) ;
#16082=ORIENTED_EDGE ( 'NONE', *, *, #4977, .T. ) ;
#16098=EDGE_LOOP ( 'NONE', ( #9681, #14673 ) ) ;
#16103=CARTESIAN_POINT ( 'NONE',  ( -26.69293917519999937, -30.50310889129999836, -48.86109741659999628 ) ) ;
#16115=EDGE_LOOP ( 'NONE', ( #25370, #3735, #24918, #10847 ) ) ;
#16122=DIRECTION ( 'NONE',  ( 1.000000000000000000, 0.000000000000000000, 0.000000000000000000 ) ) ;
#16130=ORIENTED_EDGE ( 'NONE', *, *, #23275, .T. ) ;
#16149=ADVANCED_FACE ( 'NONE', ( #3808 ), #5981, .T. ) ;
#16151=CARTESIAN_POINT ( 'NONE',  ( 31.00000000000000000, -13.00000000000000000, -4.500000000000000000 ) ) ;
#16167=ORIENTED_EDGE ( 'NONE', *, *, #27993, .F. ) ;
#16168=TOROIDAL_SURFACE ( 'NONE', #23611, 52.20000000000000284, 5.000000000000000000 ) ;
#16169=LINE ( 'NONE', #5111, #22475 ) ;
#16179=FACE_OUTER_BOUND ( 'NONE', #6971, .T. ) ;
#16181=EDGE_CURVE ( 'NONE', #1871, #7380, #16024, .T. ) ;
#16186=EDGE_CURVE ( 'NONE', #17262, #21247, #10419, .T. ) ;
#16190=DIRECTION ( 'NONE',  ( 0.4794255386042041156, 0.000000000000000000, 0.8775825618903722036 ) ) ;
#16206=CARTESIAN_POINT ( 'NONE',  ( 0.000000000000000000, -39.50000000000000000, 0.000000000000000000 ) ) ;
#16209=EDGE_LOOP ( 'NONE', ( #4840, #19447, #24211, #20139 ) ) ;
#16225=CIRCLE ( 'NONE', #25560, 55.50192378860000275 ) ;
#16239=CONICAL_SURFACE ( 'NONE', #10598, 24.40223267850002031, 0.7949521073230001456 ) ;
#16251=DIRECTION ( 'NONE',  ( 0.000000000000000000, 1.000000000000000000, 0.000000000000000000 ) ) ;
#16256=ORIENTED_EDGE ( 'NONE', *, *, #26735, .T. ) ;
#16262=ORIENTED_EDGE ( 'NONE', *, *, #3374, .T. ) ;
#16273=DIRECTION ( 'NONE',  ( 0.000000000000000000, 1.000000000000000000, 0.000000000000000000 ) ) ;
#16287=CIRCLE ( 'NONE', #20475, 0.3500000000000003664 ) ;
#16307=AXIS2_PLACEMENT_3D ( 'NONE', #6170, #4278, #19300 ) ;
#16317=EDGE_LOOP ( 'NONE', ( #27214, #1424, #9271, #2750 ) ) ;
#16319=CARTESIAN_POINT ( 'NONE',  ( 0.000000000000000000, -30.20000000000000284, 0.000000000000000000 ) ) ;
#16324=EDGE_CURVE ( 'NONE', #28714, #26809, #12877, .T. ) ;
#16326=DIRECTION ( 'NONE',  ( 0.000000000000000000, 0.000000000000000000, 1.000000000000000000 ) ) ;
#16327=ORIENTED_EDGE ( 'NONE', *, *, #20476, .F. ) ;
#16331=CARTESIAN_POINT ( 'NONE',  ( 26.60903970598167589, -15.80000000000000071, 48.70752046822583736 ) ) ;
#16334=CIRCLE ( 'NONE', #14911, 14.25000000000000000 ) ;
#16341=AXIS2_PLACEMENT_3D ( 'NONE', #18387, #11811, #188 ) ;
#16343=FACE_OUTER_BOUND ( 'NONE', #20479, .T. ) ;
#16351=EDGE_CURVE ( 'NONE', #2153, #3841, #18373, .T. ) ;
#16353=EDGE_LOOP ( 'NONE', ( #18335, #23966, #2590, #12398 ) ) ;
#16357=CIRCLE ( 'NONE', #24742, 59.04999999999999716 ) ;
#16360=DIRECTION ( 'NONE',  ( 0.4794255386042036715, 0.000000000000000000, 0.8775825618903724257 ) ) ;
#16378=AXIS2_PLACEMENT_3D ( 'NONE', #25974, #5050, #27210 ) ;
#16385=DIRECTION ( 'NONE',  ( 0.4794255386042000078, 0.000000000000000000, 0.8775825618903743131 ) ) ;
#16395=ORIENTED_EDGE ( 'NONE', *, *, #25218, .F. ) ;
#16409=VERTEX_POINT ( 'NONE', #24716 ) ;
#16416=ADVANCED_FACE ( 'NONE', ( #6646 ), #25812, .F. ) ;
#16418=VERTEX_POINT ( 'NONE', #22229 ) ;
#16419=VECTOR ( 'NONE', #27891, 1000.000000000000000 ) ;
#16433=ADVANCED_FACE ( 'NONE', ( #9554 ), #15547, .F. ) ;
#16436=AXIS2_PLACEMENT_3D ( 'NONE', #2275, #8807, #1992 ) ;
#16448=FACE_OUTER_BOUND ( 'NONE', #5085, .T. ) ;
#16452=VECTOR ( 'NONE', #7915, 999.9999999999998863 ) ;
#16459=EDGE_CURVE ( 'NONE', #9851, #1181, #7235, .T. ) ;
#16460=AXIS2_PLACEMENT_3D ( 'NONE', #23050, #5677, #22904 ) ;
#16461=DIRECTION ( 'NONE',  ( 1.000000000000000000, 0.000000000000000000, 0.000000000000000000 ) ) ;
#16471=AXIS2_PLACEMENT_3D ( 'NONE', #21698, #22280, #6250 ) ;
#16474=DIRECTION ( 'NONE',  ( 1.000000000000000000, 0.000000000000000000, 0.000000000000000000 ) ) ;
#16475=CARTESIAN_POINT ( 'NONE',  ( 4.500000000000000000, -11.00000000000000000, 50.00000000000000000 ) ) ;
#16478=ORIENTED_EDGE ( 'NONE', *, *, #16680, .F. ) ;
#16486=DIRECTION ( 'NONE',  ( 0.000000000000000000, 1.000000000000000000, 0.000000000000000000 ) ) ;
#16496=AXIS2_PLACEMENT_3D ( 'NONE', #19331, #19887, #1994 ) ;
#16498=ADVANCED_FACE ( 'NONE', ( #24560 ), #2580, .F. ) ;
#16506=DIRECTION ( 'NONE',  ( 0.000000000000000000, 1.000000000000000000, 0.000000000000000000 ) ) ;
#16509=CARTESIAN_POINT ( 'NONE',  ( 27.68682485439999752, -25.10000000000000142, 50.68039294919999804 ) ) ;
#16513=CARTESIAN_POINT ( 'NONE',  ( 25.57735248450000043, -26.54349610970000128, 46.81902967690000139 ) ) ;
#16521=CARTESIAN_POINT ( 'NONE',  ( -25.34421590619999876, -10.95575221240000019, -46.39227603280000523 ) ) ;
#16542=PRESENTATION_STYLE_ASSIGNMENT (( #23247 ) ) ;
#16546=ORIENTED_EDGE ( 'NONE', *, *, #11503, .F. ) ;
#16547=FACE_OUTER_BOUND ( 'NONE', #7990, .T. ) ;
#16554=DIRECTION ( 'NONE',  ( 0.000000000000000000, -1.000000000000000000, 0.000000000000000000 ) ) ;
#16560=ORIENTED_EDGE ( 'NONE', *, *, #6184, .F. ) ;
#16567=CARTESIAN_POINT ( 'NONE',  ( 0.000000000000000000, -10.00000000000000000, 0.000000000000000000 ) ) ;
#16568=DIRECTION ( 'NONE',  ( 0.000000000000000000, 0.000000000000000000, 1.000000000000000000 ) ) ;
#16569=ORIENTED_EDGE ( 'NONE', *, *, #20226, .T. ) ;
#16572=FACE_OUTER_BOUND ( 'NONE', #26565, .T. ) ;
#16574=CIRCLE ( 'NONE', #22147, 58.54999999999999716 ) ;
#16575=DIRECTION ( 'NONE',  ( 1.000000000000000000, 0.000000000000000000, 0.000000000000000000 ) ) ;
#16578=CARTESIAN_POINT ( 'NONE',  ( 0.000000000000000000, -12.64149019679999952, 0.000000000000000000 ) ) ;
#16591=ORIENTED_EDGE ( 'NONE', *, *, #3790, .F. ) ;
#16593=EDGE_CURVE ( 'NONE', #28180, #2258, #26751, .T. ) ;
#16597=DIRECTION ( 'NONE',  ( 0.000000000000000000, 1.000000000000000000, 0.000000000000000000 ) ) ;
#16598=ORIENTED_EDGE ( 'NONE', *, *, #456, .F. ) ;
#16604=ORIENTED_EDGE ( 'NONE', *, *, #5068, .T. ) ;
#16609=ADVANCED_FACE ( 'NONE', ( #17395 ), #23038, .F. ) ;
#16623=DIRECTION ( 'NONE',  ( 0.000000000000000000, 1.000000000000000000, 0.000000000000000000 ) ) ;
#16626=LINE ( 'NONE', #5420, #19350 ) ;
#16639=DIRECTION ( 'NONE',  ( 1.000000000000000000, 0.000000000000000000, 0.000000000000000000 ) ) ;
#16651=ORIENTED_EDGE ( 'NONE', *, *, #5538, .T. ) ;
#16660=CARTESIAN_POINT ( 'NONE',  ( 26.60903970598167589, -26.59999999999999787, 48.70752046822583736 ) ) ;
#16677=CARTESIAN_POINT ( 'NONE',  ( -28.19022166989999789, -39.75000000000000000, -51.60185463919999194 ) ) ;
#16679=FACE_OUTER_BOUND ( 'NONE', #12519, .T. ) ;
#16680=EDGE_CURVE ( 'NONE', #18617, #8439, #17900, .T. ) ;
#16707=VECTOR ( 'NONE', #10762, 1000.000000000000000 ) ;
#16710=ORIENTED_EDGE ( 'NONE', *, *, #13652, .T. ) ;
#16715=LINE ( 'NONE', #21655, #6111 ) ;
#16738=ORIENTED_EDGE ( 'NONE', *, *, #19619, .T. ) ;
#16747=ORIENTED_EDGE ( 'NONE', *, *, #8059, .T. ) ;
#16748=FACE_OUTER_BOUND ( 'NONE', #4773, .T. ) ;
#16751=EDGE_CURVE ( 'NONE', #19773, #11126, #16795, .T. ) ;
#16758=DIRECTION ( 'NONE',  ( 1.000000000000000000, 0.000000000000000000, 0.000000000000000000 ) ) ;
#16759=DIRECTION ( 'NONE',  ( 0.000000000000000000, -1.000000000000000000, 0.000000000000000000 ) ) ;
#16760=DIRECTION ( 'NONE',  ( 1.095614826932720052E-15, 0.000000000000000000, -1.000000000000000000 ) ) ;
#16768=DIRECTION ( 'NONE',  ( -0.4151946956541399669, 0.5000000000001689759, -0.7600087925152558821 ) ) ;
#16771=AXIS2_PLACEMENT_3D ( 'NONE', #265, #9107, #18008 ) ;
#16772=CARTESIAN_POINT ( 'NONE',  ( 27.59093974670000193, -39.32601556110000018, 50.50487643680000360 ) ) ;
#16787=EDGE_LOOP ( 'NONE', ( #19346, #7092 ) ) ;
#16795=LINE ( 'NONE', #16513, #11373 ) ;
#16800=LINE ( 'NONE', #18988, #16452 ) ;
#16814=AXIS2_PLACEMENT_3D ( 'NONE', #1369, #14199, #5587 ) ;
#16815=VECTOR ( 'NONE', #2861, 1000.000000000000000 ) ;
#16819=DIRECTION ( 'NONE',  ( 1.000000000000000000, 0.000000000000000000, 0.000000000000000000 ) ) ;
#16827=CARTESIAN_POINT ( 'NONE',  ( 0.000000000000000000, -2.000000000000000000, 0.000000000000000000 ) ) ;
#16829=CARTESIAN_POINT ( 'NONE',  ( 0.000000000000000000, -11.79999999999999893, 0.000000000000000000 ) ) ;
#16839=DIRECTION ( 'NONE',  ( 0.4794255386042040046, 0.000000000000000000, 0.8775825618903722036 ) ) ;
#16842=CARTESIAN_POINT ( 'NONE',  ( 0.000000000000000000, -11.85850980319999870, 0.000000000000000000 ) ) ;
#16854=LINE ( 'NONE', #3320, #18982 ) ;
#16864=APPLICATION_CONTEXT ( 'automotive_design' ) ;
#16875=DIRECTION ( 'NONE',  ( 0.000000000000000000, 1.000000000000000000, 0.000000000000000000 ) ) ;
#16884=EDGE_CURVE ( 'NONE', #16942, #13903, #14046, .T. ) ;
#16888=EDGE_CURVE ( 'NONE', #5395, #20122, #5370, .T. ) ;
#16896=DIRECTION ( 'NONE',  ( 1.000000000000000000, 0.000000000000000000, 0.000000000000000000 ) ) ;
#16920=LINE ( 'NONE', #25814, #25215 ) ;
#16922=CIRCLE ( 'NONE', #19245, 55.50192378860000275 ) ;
#16925=ORIENTED_EDGE ( 'NONE', *, *, #18804, .F. ) ;
#16928=CARTESIAN_POINT ( 'NONE',  ( 9.348798002780000616, -13.50000000000000000, 17.11285995690000306 ) ) ;
#16930=ORIENTED_EDGE ( 'NONE', *, *, #3849, .F. ) ;
#16933=CARTESIAN_POINT ( 'NONE',  ( -29.17304402409999753, -39.50000000000000000, -53.40089889099999709 ) ) ;
#16942=VERTEX_POINT ( 'NONE', #18129 ) ;
#16954=CARTESIAN_POINT ( 'NONE',  ( 0.000000000000000000, -23.00000000000000000, 0.000000000000000000 ) ) ;
#16960=AXIS2_PLACEMENT_3D ( 'NONE', #18020, #13643, #11300 ) ;
#16963=AXIS2_PLACEMENT_3D ( 'NONE', #11308, #8979, #6814 ) ;
#16971=EDGE_LOOP ( 'NONE', ( #1760, #27880, #15823, #13025 ) ) ;
#16984=DIRECTION ( 'NONE',  ( -0.000000000000000000, 1.000000000000000000, 0.000000000000000000 ) ) ;
#16987=AXIS2_PLACEMENT_3D ( 'NONE', #25970, #5994, #1239 ) ;
#16990=CARTESIAN_POINT ( 'NONE',  ( -27.68682485439999752, -31.69999999999999929, -50.68039294919999804 ) ) ;
#16999=ADVANCED_FACE ( 'NONE', ( #23783 ), #3058, .F. ) ;
#17008=EDGE_CURVE ( 'NONE', #12945, #6664, #1649, .T. ) ;
#17046=CARTESIAN_POINT ( 'NONE',  ( -26.69293917519999937, -23.30310889129999907, -48.86109741659999628 ) ) ;
#17054=ORIENTED_EDGE ( 'NONE', *, *, #503, .F. ) ;
#17070=VERTEX_POINT ( 'NONE', #8191 ) ;
#17077=DIRECTION ( 'NONE',  ( 1.000000000000000000, 0.000000000000000000, 0.000000000000000000 ) ) ;
#17095=CIRCLE ( 'NONE', #23608, 55.67692378859999991 ) ;
#17098=DIRECTION ( 'NONE',  ( 0.000000000000000000, 1.000000000000000000, 0.000000000000000000 ) ) ;
#17099=CARTESIAN_POINT ( 'NONE',  ( 0.000000000000000000, -13.50000000000000000, 0.000000000000000000 ) ) ;
#17103=ORIENTED_EDGE ( 'NONE', *, *, #13176, .F. ) ;
#17105=EDGE_CURVE ( 'NONE', #18741, #23988, #12751, .T. ) ;
#17114=CARTESIAN_POINT ( 'NONE',  ( -27.18988201479999844, -25.69844555429999744, -49.77074518290000071 ) ) ;
#17129=CARTESIAN_POINT ( 'NONE',  ( -25.57735248450000043, -37.08699221940000257, -46.81902967690000139 ) ) ;
#17133=ORIENTED_EDGE ( 'NONE', *, *, #1222, .T. ) ;
#17140=CARTESIAN_POINT ( 'NONE',  ( -27.68682485439999752, -24.80000000000000071, -50.68039294919999804 ) ) ;
#17150=DIRECTION ( 'NONE',  ( 1.000000000000000000, 0.000000000000000000, 0.000000000000000000 ) ) ;
#17176=VECTOR ( 'NONE', #17724, 999.9999999999998863 ) ;
#17200=EDGE_CURVE ( 'NONE', #22875, #23028, #736, .T. ) ;
#17207=CARTESIAN_POINT ( 'NONE',  ( 0.000000000000000000, -2.000000000000000000, 0.000000000000000000 ) ) ;
#17208=ORIENTED_EDGE ( 'NONE', *, *, #18312, .F. ) ;
#17213=EDGE_LOOP ( 'NONE', ( #10377, #18566, #20, #14649 ) ) ;
#17219=ORIENTED_EDGE ( 'NONE', *, *, #26996, .T. ) ;
#17227=DIRECTION ( 'NONE',  ( 0.000000000000000000, -1.000000000000000000, 0.000000000000000000 ) ) ;
#17237=TOROIDAL_SURFACE ( 'NONE', #8377, 55.85192378860000417, 0.3499999999999999778 ) ;
#17245=EDGE_LOOP ( 'NONE', ( #3513, #18526, #27657, #23442 ) ) ;
#17253=DIRECTION ( 'NONE',  ( 0.8775825618903722036, 0.000000000000000000, -0.4794255386042041156 ) ) ;
#17260=FACE_BOUND ( 'NONE', #14999, .T. ) ;
#17262=VERTEX_POINT ( 'NONE', #18243 ) ;
#17263=VECTOR ( 'NONE', #7575, 999.9999999999998863 ) ;
#17270=EDGE_CURVE ( 'NONE', #22334, #13365, #7031, .T. ) ;
#17271=VERTEX_POINT ( 'NONE', #25097 ) ;
#17276=( GEOMETRIC_REPRESENTATION_CONTEXT ( 3 ) GLOBAL_UNCERTAINTY_ASSIGNED_CONTEXT ( ( #10594 ) ) GLOBAL_UNIT_ASSIGNED_CONTEXT ( ( #1392, #27764, #23108 ) ) REPRESENTATION_CONTEXT ( 'NONE', 'WORKASPACE' ) );
#17280=ORIENTED_EDGE ( 'NONE', *, *, #18763, .T. ) ;
#17281=AXIS2_PLACEMENT_3D ( 'NONE', #24095, #24247, #4430 ) ;
#17290=ADVANCED_FACE ( 'NONE', ( #19233 ), #3494, .T. ) ;
#17292=CARTESIAN_POINT ( 'NONE',  ( 0.000000000000000000, -15.80000000000000071, 0.000000000000000000 ) ) ;
#17297=DIRECTION ( 'NONE',  ( 0.000000000000000000, 1.000000000000000000, 0.000000000000000000 ) ) ;
#17301=AXIS2_PLACEMENT_3D ( 'NONE', #5688, #16486, #20870 ) ;
#17303=EDGE_CURVE ( 'NONE', #20739, #16026, #250, .T. ) ;
#17305=DIRECTION ( 'NONE',  ( 0.000000000000000000, -1.000000000000000000, 0.000000000000000000 ) ) ;
#17313=CARTESIAN_POINT ( 'NONE',  ( 0.000000000000000000, -29.89689110870000022, 0.000000000000000000 ) ) ;
#17318=CIRCLE ( 'NONE', #8472, 8.099999999999999645 ) ;
#17323=CARTESIAN_POINT ( 'NONE',  ( 0.000000000000000000, -26.90310889129999694, 0.000000000000000000 ) ) ;
#17326=ADVANCED_FACE ( 'NONE', ( #1338 ), #3791, .F. ) ;
#17330=CARTESIAN_POINT ( 'NONE',  ( 0.000000000000000000, -12.64149019679999952, 0.000000000000000000 ) ) ;
#17333=CARTESIAN_POINT ( 'NONE',  ( 27.68682485439999752, -21.50000000000000000, 50.68039294919999804 ) ) ;
#17338=DIRECTION ( 'NONE',  ( 0.000000000000000000, 1.000000000000000000, 0.000000000000000000 ) ) ;
#17349=DIRECTION ( 'NONE',  ( -0.000000000000000000, 1.000000000000000000, 0.000000000000000000 ) ) ;
#17360=CARTESIAN_POINT ( 'NONE',  ( 0.000000000000000000, -13.50000000000000000, 0.000000000000000000 ) ) ;
#17361=ORIENTED_EDGE ( 'NONE', *, *, #20069, .T. ) ;
#17373=CARTESIAN_POINT ( 'NONE',  ( -29.41275679339999982, -37.50000000000000000, -53.83969017199999740 ) ) ;
#17379=VECTOR ( 'NONE', #21345, 999.9999999999998863 ) ;
#17390=CARTESIAN_POINT ( 'NONE',  ( -5.813199663199999812, -6.776234273679999198, -10.64099060729999913 ) ) ;
#17395=FACE_OUTER_BOUND ( 'NONE', #17213, .T. ) ;
#17401=DIRECTION ( 'NONE',  ( 0.000000000000000000, 1.000000000000000000, 0.000000000000000000 ) ) ;
#17402=EDGE_LOOP ( 'NONE', ( #11941, #5131, #13977, #27353 ) ) ;
#17413=DIRECTION ( 'NONE',  ( 1.000000000000000000, 0.000000000000000000, 0.000000000000000000 ) ) ;
#17422=CARTESIAN_POINT ( 'NONE',  ( 0.000000000000000000, -14.00000000000000000, 0.000000000000000000 ) ) ;
#17428=AXIS2_PLACEMENT_3D ( 'NONE', #2256, #11102, #8934 ) ;
#17430=CIRCLE ( 'NONE', #9509, 9.500000000000000000 ) ;
#17466=ORIENTED_EDGE ( 'NONE', *, *, #24925, .F. ) ;
#17476=ORIENTED_EDGE ( 'NONE', *, *, #6883, .F. ) ;
#17479=DIRECTION ( 'NONE',  ( 0.4794255386042040601, 0.000000000000000000, 0.8775825618903720926 ) ) ;
#17489=ORIENTED_EDGE ( 'NONE', *, *, #21763, .F. ) ;
#17500=AXIS2_PLACEMENT_3D ( 'NONE', #16842, #7395, #1145 ) ;
#17506=DIRECTION ( 'NONE',  ( 1.000000000000000000, 0.000000000000000000, 0.000000000000000000 ) ) ;
#17516=LINE ( 'NONE', #20536, #25639 ) ;
#17545=CARTESIAN_POINT ( 'NONE',  ( -27.68682485439999752, -21.50000000000000000, -50.68039294919999804 ) ) ;
#17559=AXIS2_PLACEMENT_3D ( 'NONE', #19100, #5961, #25808 ) ;
#17568=ADVANCED_FACE ( 'NONE', ( #19935 ), #1150, .F. ) ;
#17570=EDGE_CURVE ( 'NONE', #13393, #6364, #24465, .T. ) ;
#17596=EDGE_CURVE ( 'NONE', #1478, #20961, #24026, .T. ) ;
#17609=DIRECTION ( 'NONE',  ( 0.000000000000000000, 1.000000000000000000, 0.000000000000000000 ) ) ;
#17616=FACE_OUTER_BOUND ( 'NONE', #15280, .T. ) ;
#17622=DIRECTION ( 'NONE',  ( 0.000000000000000000, 1.000000000000000000, 0.000000000000000000 ) ) ;
#17626=DIRECTION ( 'NONE',  ( 0.000000000000000000, 1.000000000000000000, 0.000000000000000000 ) ) ;
#17629=CARTESIAN_POINT ( 'NONE',  ( 25.09792694589999940, -16.00000000000000000, 45.94144711499999545 ) ) ;
#17631=ADVANCED_FACE ( 'NONE', ( #26222 ), #27719, .F. ) ;
#17638=DIRECTION ( 'NONE',  ( 0.000000000000000000, 1.000000000000000000, 0.000000000000000000 ) ) ;
#17643=AXIS2_PLACEMENT_3D ( 'NONE', #15848, #24166, #4199 ) ;
#17648=CYLINDRICAL_SURFACE ( 'NONE', #14385, 57.74999999999999289 ) ;
#17650=ORIENTED_EDGE ( 'NONE', *, *, #1656, .T. ) ;
#17651=DIRECTION ( 'NONE',  ( 0.000000000000000000, 1.000000000000000000, 0.000000000000000000 ) ) ;
#17666=EDGE_LOOP ( 'NONE', ( #17489, #2342, #17219, #22044 ) ) ;
#17670=EDGE_CURVE ( 'NONE', #24319, #618, #17917, .T. ) ;
#17695=CARTESIAN_POINT ( 'NONE',  ( 0.000000000000000000, -34.10310889129999623, 0.000000000000000000 ) ) ;
#17703=CONICAL_SURFACE ( 'NONE', #16771, 55.67692378859999280, 1.047197551199999799 ) ;
#17704=AXIS2_PLACEMENT_3D ( 'NONE', #12667, #19524, #1766 ) ;
#17716=CARTESIAN_POINT ( 'NONE',  ( 4.500000000000000000, -15.00000000000000000, 50.00000000000000000 ) ) ;
#17720=ORIENTED_EDGE ( 'NONE', *, *, #26289, .T. ) ;
#17724=DIRECTION ( 'NONE',  ( -0.4151946956541399669, 0.5000000000001689759, -0.7600087925152558821 ) ) ;
#17731=VERTEX_POINT ( 'NONE', #11337 ) ;
#17740=ORIENTED_EDGE ( 'NONE', *, *, #14169, .T. ) ;
#17749=ORIENTED_EDGE ( 'NONE', *, *, #11503, .T. ) ;
#17751=DIRECTION ( 'NONE',  ( 0.000000000000000000, 1.000000000000000000, 0.000000000000000000 ) ) ;
#17753=EDGE_LOOP ( 'NONE', ( #5153, #27378, #11482, #28212 ) ) ;
#17767=DIRECTION ( 'NONE',  ( 0.4794255386042040601, 0.000000000000000000, 0.8775825618903720926 ) ) ;
#17775=CARTESIAN_POINT ( 'NONE',  ( -26.60903970598167589, -30.20000000000000284, -48.70752046822583736 ) ) ;
#17778=SHAPE_DEFINITION_REPRESENTATION ( #4079, #5912 ) ;
#17790=FACE_OUTER_BOUND ( 'NONE', #22188, .T. ) ;
#17800=APPLICATION_CONTEXT ( 'automotive_design' ) ;
#17808=DIRECTION ( 'NONE',  ( 0.000000000000000000, 1.000000000000000000, 0.000000000000000000 ) ) ;
#17816=FACE_OUTER_BOUND ( 'NONE', #19933, .T. ) ;
#17817=CIRCLE ( 'NONE', #23420, 55.67692378859999991 ) ;
#17823=EDGE_LOOP ( 'NONE', ( #18385, #20812, #8589, #18468 ) ) ;
#17829=VERTEX_POINT ( 'NONE', #12725 ) ;
#17859=AXIS2_PLACEMENT_3D ( 'NONE', #23672, #3716, #12577 ) ;
#17865=DIRECTION ( 'NONE',  ( 0.000000000000000000, 1.000000000000000000, 0.000000000000000000 ) ) ;
#17881=CIRCLE ( 'NONE', #9021, 55.67692378859999991 ) ;
#17890=ADVANCED_FACE ( 'NONE', ( #21777, #28472, #8510, #14776, #17260, #28055 ), #19440, .F. ) ;
#17895=DIRECTION ( 'NONE',  ( 1.000000000000000000, 0.000000000000000000, 0.000000000000000000 ) ) ;
#17896=ORIENTED_EDGE ( 'NONE', *, *, #7673, .T. ) ;
#17900=CIRCLE ( 'NONE', #5354, 57.75000000000000000 ) ;
#17902=EDGE_CURVE ( 'NONE', #23053, #18448, #23013, .T. ) ;
#17913=CARTESIAN_POINT ( 'NONE',  ( 50.00000000000000000, -13.00000000000000000, 4.500000000000000000 ) ) ;
#17916=ORIENTED_EDGE ( 'NONE', *, *, #3849, .T. ) ;
#17917=LINE ( 'NONE', #27102, #25787 ) ;
#17925=DIRECTION ( 'NONE',  ( 1.000000000000000000, 0.000000000000000000, 0.000000000000000000 ) ) ;
#17926=DIRECTION ( 'NONE',  ( 0.000000000000000000, 1.000000000000000000, 0.000000000000000000 ) ) ;
#17931=CARTESIAN_POINT ( 'NONE',  ( -31.00000000000000000, -11.00000000000000000, -4.500000000000000000 ) ) ;
#17933=DIRECTION ( 'NONE',  ( 0.4794255386042040046, 0.000000000000000000, 0.8775825618903722036 ) ) ;
#17990=DIRECTION ( 'NONE',  ( 1.000000000000000000, 0.000000000000000000, 0.000000000000000000 ) ) ;
#18008=DIRECTION ( 'NONE',  ( 0.4794255386042040046, 0.000000000000000000, 0.8775825618903722036 ) ) ;
#18011=CARTESIAN_POINT ( 'NONE',  ( 0.000000000000000000, -17.89999999999999858, 0.000000000000000000 ) ) ;
#18020=CARTESIAN_POINT ( 'NONE',  ( 0.000000000000000000, -23.30310889129999907, 0.000000000000000000 ) ) ;
#18031=EDGE_CURVE ( 'NONE', #23988, #18741, #17881, .T. ) ;
#18033=VERTEX_POINT ( 'NONE', #22958 ) ;
#18043=CARTESIAN_POINT ( 'NONE',  ( 0.000000000000000000, -16.50000000000000000, 0.000000000000000000 ) ) ;
#18056=EDGE_CURVE ( 'NONE', #26990, #13393, #691, .T. ) ;
#18060=CARTESIAN_POINT ( 'NONE',  ( 40.50000000000000000, -11.00000000000000000, 4.500000000000000000 ) ) ;
#18071=ORIENTED_EDGE ( 'NONE', *, *, #16593, .T. ) ;
#18073=FACE_OUTER_BOUND ( 'NONE', #20360, .T. ) ;
#18088=DIRECTION ( 'NONE',  ( 0.000000000000000000, 1.000000000000000000, 0.000000000000000000 ) ) ;
#18094=DIRECTION ( 'NONE',  ( 0.000000000000000000, 1.000000000000000000, 0.000000000000000000 ) ) ;
#18120=ORIENTED_EDGE ( 'NONE', *, *, #25959, .T. ) ;
#18129=CARTESIAN_POINT ( 'NONE',  ( -26.69293917519999937, -29.89689110870000022, -48.86109741659999628 ) ) ;
#18153=DIRECTION ( 'NONE',  ( 0.000000000000000000, 1.000000000000000000, 0.000000000000000000 ) ) ;
#18154=DIRECTION ( 'NONE',  ( 0.000000000000000000, 1.000000000000000000, 0.000000000000000000 ) ) ;
#18156=CARTESIAN_POINT ( 'NONE',  ( 0.000000000000000000, -12.64149019679999952, 0.000000000000000000 ) ) ;
#18168=EDGE_LOOP ( 'NONE', ( #16598, #1457, #19213, #975 ) ) ;
#18169=TOROIDAL_SURFACE ( 'NONE', #26542, 60.85000000000000142, 0.5000000000000000000 ) ;
#18185=PLANE ( 'NONE',  #7124 ) ;
#18198=EDGE_LOOP ( 'NONE', ( #16043, #4820, #6480, #20377 ) ) ;
#18199=CARTESIAN_POINT ( 'NONE',  ( 11.87191034930000022, -15.14308496720000008, 21.73138612759999688 ) ) ;
#18238=EDGE_CURVE ( 'NONE', #15673, #25924, #19669, .T. ) ;
#18243=CARTESIAN_POINT ( 'NONE',  ( 3.883346862689999845, -16.50000000000000000, 7.108418751309999450 ) ) ;
#18246=CARTESIAN_POINT ( 'NONE',  ( -27.68682485439999752, -17.30000000000000071, -50.68039294919999804 ) ) ;
#18248=CIRCLE ( 'NONE', #16436, 8.099999999999999645 ) ;
#18274=ADVANCED_FACE ( 'NONE', ( #8324 ), #7620, .F. ) ;
#18276=CIRCLE ( 'NONE', #4774, 0.3500000000000003664 ) ;
#18277=CARTESIAN_POINT ( 'NONE',  ( -29.41275679339999982, -25.00000000000000000, -53.83969017199999740 ) ) ;
#18285=ORIENTED_EDGE ( 'NONE', *, *, #4711, .T. ) ;
#18293=COLOUR_RGB ( '', 0.66274510, 0.83137255, 0.94901961) ;
#18297=DIRECTION ( 'NONE',  ( 0.000000000000000000, -1.000000000000000000, 0.000000000000000000 ) ) ;
#18312=EDGE_CURVE ( 'NONE', #103, #6607, #27625, .T. ) ;
#18331=ORIENTED_EDGE ( 'NONE', *, *, #22245, .F. ) ;
#18335=ORIENTED_EDGE ( 'NONE', *, *, #9964, .F. ) ;
#18336=AXIS2_PLACEMENT_3D ( 'NONE', #5540, #12230, #23184 ) ;
#18338=FACE_OUTER_BOUND ( 'NONE', #28172, .T. ) ;
#18352=AXIS2_PLACEMENT_3D ( 'NONE', #5617, #21217, #16839 ) ;
#18373=CIRCLE ( 'NONE', #16496, 55.50192378860000275 ) ;
#18375=CARTESIAN_POINT ( 'NONE',  ( 26.77683864449999973, -15.80000000000000071, 49.01467436490000296 ) ) ;
#18378=ADVANCED_FACE ( 'NONE', ( #2813 ), #28510, .T. ) ;
#18385=ORIENTED_EDGE ( 'NONE', *, *, #15396, .T. ) ;
#18387=CARTESIAN_POINT ( 'NONE',  ( -26.77683864449999973, -26.59999999999999787, -49.01467436490000296 ) ) ;
#18389=ORIENTED_EDGE ( 'NONE', *, *, #2721, .T. ) ;
#18391=CARTESIAN_POINT ( 'NONE',  ( 0.000000000000000000, -12.64149019679999952, 0.000000000000000000 ) ) ;
#18393=ORIENTED_EDGE ( 'NONE', *, *, #15947, .F. ) ;
#18398=CARTESIAN_POINT ( 'NONE',  ( -26.77683864449999973, -15.80000000000000071, -49.01467436490000296 ) ) ;
#18401=ADVANCED_FACE ( 'NONE', ( #26997 ), #13160, .T. ) ;
#18403=ORIENTED_EDGE ( 'NONE', *, *, #20275, .F. ) ;
#18406=CONICAL_SURFACE ( 'NONE', #11894, 58.55000000000003979, 0.7853981633970000820 ) ;
#18446=DIRECTION ( 'NONE',  ( 0.000000000000000000, -1.000000000000000000, 0.000000000000000000 ) ) ;
#18448=VERTEX_POINT ( 'NONE', #12652 ) ;
#18459=FACE_OUTER_BOUND ( 'NONE', #15517, .T. ) ;
#18461=ORIENTED_EDGE ( 'NONE', *, *, #352, .T. ) ;
#18468=ORIENTED_EDGE ( 'NONE', *, *, #23659, .F. ) ;
#18470=EDGE_CURVE ( 'NONE', #6607, #103, #12671, .T. ) ;
#18472=EDGE_CURVE ( 'NONE', #8384, #4012, #23607, .T. ) ;
#18477=ORIENTED_EDGE ( 'NONE', *, *, #157, .F. ) ;
#18499=CARTESIAN_POINT ( 'NONE',  ( 28.07036528529999941, -39.41300778060000454, 51.38245899869999533 ) ) ;
#18501=EDGE_LOOP ( 'NONE', ( #4931, #20705, #26941, #21585 ) ) ;
#18511=AXIS2_PLACEMENT_3D ( 'NONE', #10378, #19295, #14898 ) ;
#18513=VERTEX_POINT ( 'NONE', #27846 ) ;
#18519=ORIENTED_EDGE ( 'NONE', *, *, #357, .T. ) ;
#18520=LINE ( 'NONE', #5816, #5980 ) ;
#18521=CARTESIAN_POINT ( 'NONE',  ( 27.18988201479999844, -32.89844555429999673, 49.77074518290000071 ) ) ;
#18526=ORIENTED_EDGE ( 'NONE', *, *, #6204, .F. ) ;
#18533=DIRECTION ( 'NONE',  ( 0.4794255386042041156, 0.000000000000000000, 0.8775825618903720926 ) ) ;
#18534=FACE_OUTER_BOUND ( 'NONE', #3605, .T. ) ;
#18547=CARTESIAN_POINT ( 'NONE',  ( 0.000000000000000000, -2.000000000000000000, 0.000000000000000000 ) ) ;
#18560=EDGE_LOOP ( 'NONE', ( #19180, #21452, #1274, #12895 ) ) ;
#18566=ORIENTED_EDGE ( 'NONE', *, *, #21671, .T. ) ;
#18569=CARTESIAN_POINT ( 'NONE',  ( 27.18988201479999844, -34.70155444569999759, 49.77074518290000071 ) ) ;
#18577=TOROIDAL_SURFACE ( 'NONE', #10152, 55.85192378860000417, 0.3499999999999999778 ) ;
#18586=DIRECTION ( 'NONE',  ( 0.8775825618903722036, 0.000000000000000000, -0.4794255386042041156 ) ) ;
#18592=CARTESIAN_POINT ( 'NONE',  ( 0.000000000000000000, -37.50000000000000000, 0.000000000000000000 ) ) ;
#18607=DIRECTION ( 'NONE',  ( 1.000000000000000000, 0.000000000000000000, 0.000000000000000000 ) ) ;
#18611=DIRECTION ( 'NONE',  ( 1.000000000000000000, 0.000000000000000000, 0.000000000000000000 ) ) ;
#18617=VERTEX_POINT ( 'NONE', #15565 ) ;
#18619=VECTOR ( 'NONE', #872, 1000.000000000000000 ) ;
#18620=CARTESIAN_POINT ( 'NONE',  ( 27.68682485439999752, -28.69999999999999929, 50.68039294919999804 ) ) ;
#18623=EDGE_LOOP ( 'NONE', ( #15064, #15761 ) ) ;
#18642=ORIENTED_EDGE ( 'NONE', *, *, #8427, .T. ) ;
#18644=EDGE_CURVE ( 'NONE', #6664, #23028, #17817, .T. ) ;
#18657=CIRCLE ( 'NONE', #11159, 58.54999999999999716 ) ;
#18662=CIRCLE ( 'NONE', #13988, 2.999999999999998224 ) ;
#18663=CARTESIAN_POINT ( 'NONE',  ( 25.09792694589999940, -15.00000000000000000, 45.94144711499999545 ) ) ;
#18670=CARTESIAN_POINT ( 'NONE',  ( 4.500000000000000000, -11.00000000000000000, -50.00000000000000000 ) ) ;
#18679=CARTESIAN_POINT ( 'NONE',  ( -4.500000000000000000, -12.50000000000000000, 40.50000000000000000 ) ) ;
#18690=FACE_OUTER_BOUND ( 'NONE', #5469, .T. ) ;
#18692=AXIS2_PLACEMENT_3D ( 'NONE', #4459, #13633, #9110 ) ;
#18697=DIRECTION ( 'NONE',  ( 0.000000000000000000, 1.000000000000000000, 0.000000000000000000 ) ) ;
#18699=AXIS2_PLACEMENT_3D ( 'NONE', #26578, #2115, #15330 ) ;
#18706=CARTESIAN_POINT ( 'NONE',  ( 0.000000000000000000, -10.50000000000000000, 0.000000000000000000 ) ) ;
#18715=CARTESIAN_POINT ( 'NONE',  ( -29.41275679339999982, -11.79999999999999893, -53.83969017199999740 ) ) ;
#18725=CIRCLE ( 'NONE', #17301, 55.50192378860000275 ) ;
#18735=DIRECTION ( 'NONE',  ( -0.8775825618903722036, 0.000000000000000000, 0.4794255386042041156 ) ) ;
#18741=VERTEX_POINT ( 'NONE', #16103 ) ;
#18748=LINE ( 'NONE', #20794, #21533 ) ;
#18750=CARTESIAN_POINT ( 'NONE',  ( 0.000000000000000000, -37.57799544290000426, 0.000000000000000000 ) ) ;
#18751=PLANE ( 'NONE',  #24386 ) ;
#18755=DIRECTION ( 'NONE',  ( 0.000000000000000000, 1.000000000000000000, 0.000000000000000000 ) ) ;
#18760=AXIS2_PLACEMENT_3D ( 'NONE', #27448, #2975, #7493 ) ;
#18761=ORIENTED_EDGE ( 'NONE', *, *, #9705, .T. ) ;
#18763=EDGE_CURVE ( 'NONE', #19846, #3448, #18748, .T. ) ;
#18771=DIRECTION ( 'NONE',  ( 1.000000000000000000, 0.000000000000000000, 0.000000000000000000 ) ) ;
#18775=CARTESIAN_POINT ( 'NONE',  ( -10.54736184929999965, -12.25000000000000000, -19.30681636159999925 ) ) ;
#18776=CARTESIAN_POINT ( 'NONE',  ( 0.000000000000000000, -15.80000000000000071, 0.000000000000000000 ) ) ;
#18779=DIRECTION ( 'NONE',  ( 0.000000000000000000, 1.000000000000000000, 0.000000000000000000 ) ) ;
#18782=AXIS2_PLACEMENT_3D ( 'NONE', #1228, #5577, #21038 ) ;
#18790=DIRECTION ( 'NONE',  ( 1.000000000000000000, 0.000000000000000000, 0.000000000000000000 ) ) ;
#18793=ORIENTED_EDGE ( 'NONE', *, *, #15543, .F. ) ;
#18799=EDGE_LOOP ( 'NONE', ( #11476, #172, #3001, #422 ) ) ;
#18802=VECTOR ( 'NONE', #15286, 1000.000000000000114 ) ;
#18804=EDGE_CURVE ( 'NONE', #3592, #5336, #4333, .T. ) ;
#18807=EDGE_LOOP ( 'NONE', ( #4325, #3555, #20977, #3435 ) ) ;
#18815=CONICAL_SURFACE ( 'NONE', #6219, 55.67692378859999280, 1.047197551199999799 ) ;
#18820=ORIENTED_EDGE ( 'NONE', *, *, #5933, .F. ) ;
#18826=AXIS2_PLACEMENT_3D ( 'NONE', #3786, #11017, #17767 ) ;
#18829=ORIENTED_EDGE ( 'NONE', *, *, #13232, .F. ) ;
#18834=CARTESIAN_POINT ( 'NONE',  ( 0.000000000000000000, -14.30000000000000071, 0.000000000000000000 ) ) ;
#18841=ORIENTED_EDGE ( 'NONE', *, *, #8798, .F. ) ;
#18845=DIRECTION ( 'NONE',  ( 0.4794255386042040046, 0.000000000000000000, 0.8775825618903722036 ) ) ;
#18856=ORIENTED_EDGE ( 'NONE', *, *, #4711, .F. ) ;
#18862=DIRECTION ( 'NONE',  ( 0.000000000000000000, 1.000000000000000000, 0.000000000000000000 ) ) ;
#18866=DIRECTION ( 'NONE',  ( 0.000000000000000000, 1.000000000000000000, 0.000000000000000000 ) ) ;
#18867=ORIENTED_EDGE ( 'NONE', *, *, #2050, .T. ) ;
#18870=VECTOR ( 'NONE', #23454, 1000.000000000000000 ) ;
#18871=EDGE_CURVE ( 'NONE', #28370, #25772, #1567, .T. ) ;
#18880=EDGE_LOOP ( 'NONE', ( #599, #19315, #26497, #21605 ) ) ;
#18882=CARTESIAN_POINT ( 'NONE',  ( 31.00000000000000000, -15.00000000000000000, -4.500000000000000000 ) ) ;
#18902=EDGE_CURVE ( 'NONE', #19419, #640, #19161, .T. ) ;
#18904=EDGE_CURVE ( 'NONE', #15453, #258, #25996, .T. ) ;
#18909=ORIENTED_EDGE ( 'NONE', *, *, #5573, .T. ) ;
#18913=DIRECTION ( 'NONE',  ( 0.4794255386042000078, 0.000000000000000000, 0.8775825618903743131 ) ) ;
#18933=ORIENTED_EDGE ( 'NONE', *, *, #8902, .T. ) ;
#18948=DIRECTION ( 'NONE',  ( 0.000000000000000000, 1.000000000000000000, 0.000000000000000000 ) ) ;
#18967=DIRECTION ( 'NONE',  ( -0.8775825618903722036, 0.000000000000000000, 0.4794255386042041156 ) ) ;
#18969=ORIENTED_EDGE ( 'NONE', *, *, #21053, .F. ) ;
#18973=ORIENTED_EDGE ( 'NONE', *, *, #10586, .T. ) ;
#18979=DIRECTION ( 'NONE',  ( -1.000000000000000000, 0.000000000000000000, -1.095614826932720052E-15 ) ) ;
#18982=VECTOR ( 'NONE', #25881, 1000.000000000000000 ) ;
#18984=CARTESIAN_POINT ( 'NONE',  ( 10.54736184929999965, -12.25000000000000000, 19.30681636159999925 ) ) ;
#18988=CARTESIAN_POINT ( 'NONE',  ( -27.18988201479999844, -23.90155444570000043, -49.77074518290000071 ) ) ;
#18989=EDGE_CURVE ( 'NONE', #6736, #731, #2995, .T. ) ;
#18999=EDGE_CURVE ( 'NONE', #8881, #5109, #22512, .T. ) ;
#19005=AXIS2_PLACEMENT_3D ( 'NONE', #4646, #307, #13676 ) ;
#19009=AXIS2_PLACEMENT_3D ( 'NONE', #11013, #21555, #24314 ) ;
#19014=DIRECTION ( 'NONE',  ( 1.000000000000000000, 0.000000000000000000, 0.000000000000000000 ) ) ;
#19024=EDGE_CURVE ( 'NONE', #25924, #15673, #16922, .T. ) ;
#19044=AXIS2_PLACEMENT_3D ( 'NONE', #15466, #22056, #6308 ) ;
#19047=CARTESIAN_POINT ( 'NONE',  ( 40.50000000000000000, -12.50000000000000000, -4.500000000000000000 ) ) ;
#19048=ORIENTED_EDGE ( 'NONE', *, *, #12704, .F. ) ;
#19056=EDGE_CURVE ( 'NONE', #26186, #14188, #26705, .T. ) ;
#19061=CARTESIAN_POINT ( 'NONE',  ( 0.000000000000000000, -30.20000000000000284, 0.000000000000000000 ) ) ;
#19066=AXIS2_PLACEMENT_3D ( 'NONE', #16567, #8101, #5904 ) ;
#19067=AXIS2_PLACEMENT_3D ( 'NONE', #27020, #2398, #7063 ) ;
#19078=EDGE_LOOP ( 'NONE', ( #22742, #360, #3468, #8511 ) ) ;
#19082=DIRECTION ( 'NONE',  ( -0.000000000000000000, 1.000000000000000000, 0.000000000000000000 ) ) ;
#19084=AXIS2_PLACEMENT_3D ( 'NONE', #21297, #23074, #3119 ) ;
#19100=CARTESIAN_POINT ( 'NONE',  ( 0.000000000000000000, -16.10310889129999623, 0.000000000000000000 ) ) ;
#19105=CIRCLE ( 'NONE', #3742, 12.25068835559999947 ) ;
#19106=CIRCLE ( 'NONE', #6533, 55.67692378859999991 ) ;
#19161=LINE ( 'NONE', #12433, #17379 ) ;
#19176=AXIS2_PLACEMENT_3D ( 'NONE', #8577, #24178, #8707 ) ;
#19180=ORIENTED_EDGE ( 'NONE', *, *, #2412, .F. ) ;
#19192=CARTESIAN_POINT ( 'NONE',  ( 0.000000000000000000, -31.69999999999999929, 0.000000000000000000 ) ) ;
#19194=AXIS2_PLACEMENT_3D ( 'NONE', #1732, #28524, #19488 ) ;
#19213=ORIENTED_EDGE ( 'NONE', *, *, #5013, .T. ) ;
#19215=TOROIDAL_SURFACE ( 'NONE', #8054, 55.85192378860000417, 0.3499999999999999778 ) ;
#19218=EDGE_CURVE ( 'NONE', #4674, #28301, #16800, .T. ) ;
#19233=FACE_OUTER_BOUND ( 'NONE', #1668, .T. ) ;
#19240=EDGE_LOOP ( 'NONE', ( #15252, #5102, #12466, #21572 ) ) ;
#19245=AXIS2_PLACEMENT_3D ( 'NONE', #2396, #17401, #20158 ) ;
#19249=EDGE_CURVE ( 'NONE', #2258, #17070, #20164, .T. ) ;
#19254=DIRECTION ( 'NONE',  ( 1.000000000000000000, 0.000000000000000000, 0.000000000000000000 ) ) ;
#19265=DIRECTION ( 'NONE',  ( 0.000000000000000000, 1.000000000000000000, 0.000000000000000000 ) ) ;
#19268=AXIS2_PLACEMENT_3D ( 'NONE', #28329, #16984, #17413 ) ;
#19285=DIRECTION ( 'NONE',  ( -0.8775825618903722036, 0.000000000000000000, 0.4794255386042041156 ) ) ;
#19290=LINE ( 'NONE', #15029, #25282 ) ;
#19291=CARTESIAN_POINT ( 'NONE',  ( 0.000000000000000000, -39.50000000000000000, 0.000000000000000000 ) ) ;
#19295=DIRECTION ( 'NONE',  ( 0.000000000000000000, 1.000000000000000000, 0.000000000000000000 ) ) ;
#19296=DIRECTION ( 'NONE',  ( 1.000000000000000000, 0.000000000000000000, 0.000000000000000000 ) ) ;
#19298=ORIENTED_EDGE ( 'NONE', *, *, #18644, .T. ) ;
#19300=DIRECTION ( 'NONE',  ( 0.4794255386042036715, 0.000000000000000000, 0.8775825618903724257 ) ) ;
#19315=ORIENTED_EDGE ( 'NONE', *, *, #21067, .F. ) ;
#19317=ADVANCED_FACE ( 'NONE', ( #21729 ), #28534, .F. ) ;
#19322=DIRECTION ( 'NONE',  ( 0.4794255386042036715, 0.000000000000000000, 0.8775825618903724257 ) ) ;
#19324=DIRECTION ( 'NONE',  ( 1.000000000000000000, 0.000000000000000000, 0.000000000000000000 ) ) ;
#19327=EDGE_LOOP ( 'NONE', ( #15035, #26531, #4417, #12726 ) ) ;
#19331=CARTESIAN_POINT ( 'NONE',  ( 0.000000000000000000, -15.80000000000000071, 0.000000000000000000 ) ) ;
#19346=ORIENTED_EDGE ( 'NONE', *, *, #5830, .F. ) ;
#19348=EDGE_CURVE ( 'NONE', #21477, #103, #5650, .T. ) ;
#19350=VECTOR ( 'NONE', #9343, 1000.000000000000000 ) ;
#19353=DIRECTION ( 'NONE',  ( -0.4151946956541399669, 0.5000000000001689759, -0.7600087925152558821 ) ) ;
#19354=ORIENTED_EDGE ( 'NONE', *, *, #26735, .F. ) ;
#19388=DIRECTION ( 'NONE',  ( 1.000000000000000000, 0.000000000000000000, 0.000000000000000000 ) ) ;
#19399=ADVANCED_FACE ( 'NONE', ( #8114 ), #21517, .T. ) ;
#19401=LINE ( 'NONE', #14605, #28317 ) ;
#19419=VERTEX_POINT ( 'NONE', #10840 ) ;
#19424=FACE_OUTER_BOUND ( 'NONE', #22644, .T. ) ;
#19426=VERTEX_POINT ( 'NONE', #15363 ) ;
#19440=PLANE ( 'NONE',  #19268 ) ;
#19441=ORIENTED_EDGE ( 'NONE', *, *, #2371, .F. ) ;
#19447=ORIENTED_EDGE ( 'NONE', *, *, #25450, .F. ) ;
#19457=ORIENTED_EDGE ( 'NONE', *, *, #17270, .F. ) ;
#19465=DIRECTION ( 'NONE',  ( 0.4794255386042036715, 0.000000000000000000, 0.8775825618903724257 ) ) ;
#19469=ORIENTED_EDGE ( 'NONE', *, *, #3466, .T. ) ;
#19488=DIRECTION ( 'NONE',  ( 1.000000000000000000, 0.000000000000000000, 0.000000000000000000 ) ) ;
#19490=VECTOR ( 'NONE', #2806, 1000.000000000000000 ) ;
#19497=ADVANCED_FACE ( 'NONE', ( #9405 ), #12021, .F. ) ;
#19503=ORIENTED_EDGE ( 'NONE', *, *, #10120, .F. ) ;
#19509=DIRECTION ( 'NONE',  ( 1.000000000000000000, 0.000000000000000000, 0.000000000000000000 ) ) ;
#19513=CYLINDRICAL_SURFACE ( 'NONE', #9338, 8.099999999999997868 ) ;
#19514=AXIS2_PLACEMENT_3D ( 'NONE', #22333, #26854, #9503 ) ;
#19515=AXIS2_PLACEMENT_3D ( 'NONE', #581, #9426, #22854 ) ;
#19524=DIRECTION ( 'NONE',  ( -0.8775825618903722036, 0.000000000000000000, 0.4794255386042041156 ) ) ;
#19525=CARTESIAN_POINT ( 'NONE',  ( -27.68682485439999752, -24.80000000000000071, -50.68039294919999804 ) ) ;
#19531=ORIENTED_EDGE ( 'NONE', *, *, #18644, .F. ) ;
#19532=ADVANCED_FACE ( 'NONE', ( #18459 ), #18751, .T. ) ;
#19541=CARTESIAN_POINT ( 'NONE',  ( 27.18988201479999844, -14.89844555430000028, 49.77074518290000071 ) ) ;
#19544=AXIS2_PLACEMENT_3D ( 'NONE', #9793, #12115, #18845 ) ;
#19548=DIRECTION ( 'NONE',  ( 0.000000000000000000, 1.000000000000000000, 0.000000000000000000 ) ) ;
#19554=ORIENTED_EDGE ( 'NONE', *, *, #2629, .F. ) ;
#19563=CIRCLE ( 'NONE', #24700, 55.67692378859999991 ) ;
#19567=LINE ( 'NONE', #17390, #9161 ) ;
#19576=FACE_OUTER_BOUND ( 'NONE', #4337, .T. ) ;
#19578=ORIENTED_EDGE ( 'NONE', *, *, #24680, .T. ) ;
#19581=CARTESIAN_POINT ( 'NONE',  ( -4.500000000000000000, -11.00000000000000000, -31.00000000000000000 ) ) ;
#19585=CONICAL_SURFACE ( 'NONE', #15357, 55.67692378859999280, 1.047197551199999799 ) ;
#19586=ORIENTED_EDGE ( 'NONE', *, *, #13312, .T. ) ;
#19587=CIRCLE ( 'NONE', #12585, 55.67692378859999991 ) ;
#19594=CARTESIAN_POINT ( 'NONE',  ( 50.00000000000000000, -11.00000000000000000, -4.500000000000000000 ) ) ;
#19596=EDGE_CURVE ( 'NONE', #19426, #24400, #23901, .T. ) ;
#19606=EDGE_CURVE ( 'NONE', #19954, #13987, #3892, .T. ) ;
#19611=DIRECTION ( 'NONE',  ( 0.000000000000000000, -1.000000000000000000, 0.000000000000000000 ) ) ;
#19612=DIRECTION ( 'NONE',  ( 0.000000000000000000, 1.000000000000000000, 0.000000000000000000 ) ) ;
#19617=DIRECTION ( 'NONE',  ( 0.4794255386042041156, 0.000000000000000000, 0.8775825618903720926 ) ) ;
#19619=EDGE_CURVE ( 'NONE', #20652, #20846, #27913, .T. ) ;
#19645=VERTEX_POINT ( 'NONE', #12854 ) ;
#19647=ADVANCED_FACE ( 'NONE', ( #23401 ), #3016, .T. ) ;
#19657=EDGE_CURVE ( 'NONE', #22334, #28503, #24855, .T. ) ;
#19669=CIRCLE ( 'NONE', #4804, 55.50192378860000275 ) ;
#19671=DIRECTION ( 'NONE',  ( 0.000000000000000000, 1.000000000000000000, 0.000000000000000000 ) ) ;
#19681=CIRCLE ( 'NONE', #7149, 0.3500000000000003664 ) ;
#19682=CARTESIAN_POINT ( 'NONE',  ( 4.500000000000000000, -13.00000000000000000, -31.00000000000000000 ) ) ;
#19696=AXIS2_PLACEMENT_3D ( 'NONE', #6280, #15851, #24904 ) ;
#19711=EDGE_LOOP ( 'NONE', ( #5127, #15468, #1449, #3222 ) ) ;
#19734=VECTOR ( 'NONE', #6496, 1000.000000000000000 ) ;
#19737=CARTESIAN_POINT ( 'NONE',  ( 0.000000000000000000, -33.79999999999999716, 0.000000000000000000 ) ) ;
#19745=CONICAL_SURFACE ( 'NONE', #27205, 57.74999999999999289, 1.152571997220000144 ) ;
#19747=FACE_BOUND ( 'NONE', #12876, .T. ) ;
#19769=DIRECTION ( 'NONE',  ( 0.000000000000000000, 1.000000000000000000, 0.000000000000000000 ) ) ;
#19773=VERTEX_POINT ( 'NONE', #24689 ) ;
#19786=DIRECTION ( 'NONE',  ( 0.4794255386042036715, 0.000000000000000000, 0.8775825618903724257 ) ) ;
#19787=CARTESIAN_POINT ( 'NONE',  ( 26.72663706610000034, -37.96100227850000408, 48.92278099219999632 ) ) ;
#19794=DIRECTION ( 'NONE',  ( 0.8775825618903722036, 0.000000000000000000, -0.4794255386042041156 ) ) ;
#19798=DIRECTION ( 'NONE',  ( 0.000000000000000000, 1.000000000000000000, 0.000000000000000000 ) ) ;
#19801=CARTESIAN_POINT ( 'NONE',  ( 25.81706525379999917, -37.08699221940000257, 47.25782095779999992 ) ) ;
#19829=CARTESIAN_POINT ( 'NONE',  ( 0.000000000000000000, -2.000000000000000000, 0.000000000000000000 ) ) ;
#19836=CARTESIAN_POINT ( 'NONE',  ( 0.000000000000000000, -33.49689110869999809, 0.000000000000000000 ) ) ;
#19846=VERTEX_POINT ( 'NONE', #5094 ) ;
#19849=ADVANCED_FACE ( 'NONE', ( #16011 ), #18815, .T. ) ;
#19855=ORIENTED_EDGE ( 'NONE', *, *, #9637, .F. ) ;
#19870=AXIS2_PLACEMENT_3D ( 'NONE', #19879, #15504, #24413 ) ;
#19871=ORIENTED_EDGE ( 'NONE', *, *, #6184, .T. ) ;
#19879=CARTESIAN_POINT ( 'NONE',  ( -26.77683864449999973, -19.40000000000000213, -49.01467436490000296 ) ) ;
#19885=ADVANCED_FACE ( 'NONE', ( #11023 ), #2774, .T. ) ;
#19887=DIRECTION ( 'NONE',  ( 0.000000000000000000, 1.000000000000000000, 0.000000000000000000 ) ) ;
#19891=EDGE_CURVE ( 'NONE', #2012, #1944, #13201, .T. ) ;
#19896=EDGE_LOOP ( 'NONE', ( #28353, #7914, #22823, #16395 ) ) ;
#19911=ORIENTED_EDGE ( 'NONE', *, *, #18871, .T. ) ;
#19912=CYLINDRICAL_SURFACE ( 'NONE', #3311, 53.34999999999998721 ) ;
#19914=ORIENTED_EDGE ( 'NONE', *, *, #21358, .T. ) ;
#19933=EDGE_LOOP ( 'NONE', ( #4413, #2165, #12956, #23950 ) ) ;
#19935=FACE_OUTER_BOUND ( 'NONE', #21480, .T. ) ;
#19942=ORIENTED_EDGE ( 'NONE', *, *, #9195, .F. ) ;
#19943=DIRECTION ( 'NONE',  ( 0.4794255386042033384, 0.000000000000000000, 0.8775825618903726477 ) ) ;
#19945=VERTEX_POINT ( 'NONE', #17775 ) ;
#19950=CIRCLE ( 'NONE', #9735, 25.11294200180000047 ) ;
#19953=CIRCLE ( 'NONE', #7437, 21.60095686220000033 ) ;
#19954=VERTEX_POINT ( 'NONE', #15711 ) ;
#19963=ADVANCED_FACE ( 'NONE', ( #2330 ), #17237, .F. ) ;
#19964=DIRECTION ( 'NONE',  ( 0.4794255386042036715, 0.000000000000000000, 0.8775825618903724257 ) ) ;
#19968=ORIENTED_EDGE ( 'NONE', *, *, #12863, .F. ) ;
#20005=CARTESIAN_POINT ( 'NONE',  ( 27.68682485439999752, -28.10000000000000142, 50.68039294919999804 ) ) ;
#20021=AXIS2_PLACEMENT_3D ( 'NONE', #26972, #22295, #15720 ) ;
#20024=CIRCLE ( 'NONE', #24215, 59.04999999999999716 ) ;
#20039=VERTEX_POINT ( 'NONE', #27813 ) ;
#20043=DIRECTION ( 'NONE',  ( 0.000000000000000000, 1.000000000000000000, 0.000000000000000000 ) ) ;
#20045=CIRCLE ( 'NONE', #10256, 57.75000000000000000 ) ;
#20055=DIRECTION ( 'NONE',  ( 0.000000000000000000, 0.000000000000000000, 1.000000000000000000 ) ) ;
#20062=EDGE_LOOP ( 'NONE', ( #24901, #7453, #2746, #9149 ) ) ;
#20064=FACE_OUTER_BOUND ( 'NONE', #2577, .T. ) ;
#20066=CIRCLE ( 'NONE', #4233, 19.50000000000000000 ) ;
#20069=EDGE_CURVE ( 'NONE', #10652, #20846, #9311, .T. ) ;
#20071=AXIS2_PLACEMENT_3D ( 'NONE', #27554, #9462, #16461 ) ;
#20090=CARTESIAN_POINT ( 'NONE',  ( 0.000000000000000000, -28.69999999999999929, 0.000000000000000000 ) ) ;
#20103=CARTESIAN_POINT ( 'NONE',  ( 5.753106463249999969, -2.000000000000000000, 10.53099074269999846 ) ) ;
#20109=DIRECTION ( 'NONE',  ( 0.4794255386042037270, 0.000000000000000000, 0.8775825618903724257 ) ) ;
#20119=CARTESIAN_POINT ( 'NONE',  ( 26.69293917519999937, -34.10310889129999623, 48.86109741659999628 ) ) ;
#20122=VERTEX_POINT ( 'NONE', #5245 ) ;
#20133=AXIS2_PLACEMENT_3D ( 'NONE', #5401, #5535, #7868 ) ;
#20137=EDGE_CURVE ( 'NONE', #584, #12535, #18657, .T. ) ;
#20139=ORIENTED_EDGE ( 'NONE', *, *, #12139, .T. ) ;
#20144=EDGE_LOOP ( 'NONE', ( #25189, #21151, #15215, #16327 ) ) ;
#20148=ORIENTED_EDGE ( 'NONE', *, *, #15189, .T. ) ;
#20158=DIRECTION ( 'NONE',  ( 0.000000000000000000, 0.000000000000000000, 1.000000000000000000 ) ) ;
#20164=CIRCLE ( 'NONE', #19696, 24.50000000000000000 ) ;
#20165=FACE_OUTER_BOUND ( 'NONE', #27522, .T. ) ;
#20167=DIRECTION ( 'NONE',  ( 0.000000000000000000, 0.000000000000000000, 1.000000000000000000 ) ) ;
#20171=ADVANCED_FACE ( 'NONE', ( #22977 ), #15839, .T. ) ;
#20174=ADVANCED_FACE ( 'NONE', ( #6797 ), #27012, .T. ) ;
#20178=CYLINDRICAL_SURFACE ( 'NONE', #10308, 57.74999999999999289 ) ;
#20192=FACE_OUTER_BOUND ( 'NONE', #10020, .T. ) ;
#20194=AXIS2_PLACEMENT_3D ( 'NONE', #13716, #7474, #4681 ) ;
#20195=LINE ( 'NONE', #26768, #2389 ) ;
#20207=AXIS2_PLACEMENT_3D ( 'NONE', #28412, #26093, #1640 ) ;
#20214=ORIENTED_EDGE ( 'NONE', *, *, #24925, .T. ) ;
#20226=EDGE_CURVE ( 'NONE', #25155, #19945, #12119, .T. ) ;
#20231=FACE_OUTER_BOUND ( 'NONE', #6047, .T. ) ;
#20247=CARTESIAN_POINT ( 'NONE',  ( 0.000000000000000000, -29.89689110870000022, 0.000000000000000000 ) ) ;
#20250=AXIS2_PLACEMENT_3D ( 'NONE', #21015, #23745, #10319 ) ;
#20257=ORIENTED_EDGE ( 'NONE', *, *, #18999, .F. ) ;
#20267=DIRECTION ( 'NONE',  ( 0.000000000000000000, 1.000000000000000000, 0.000000000000000000 ) ) ;
#20275=EDGE_CURVE ( 'NONE', #21532, #13393, #3309, .T. ) ;
#20297=EDGE_CURVE ( 'NONE', #3752, #20553, #7001, .T. ) ;
#20307=FACE_OUTER_BOUND ( 'NONE', #21969, .T. ) ;
#20309=CIRCLE ( 'NONE', #13795, 55.67692378859999991 ) ;
#20315=DIRECTION ( 'NONE',  ( 1.000000000000000000, 0.000000000000000000, 0.000000000000000000 ) ) ;
#20316=ADVANCED_FACE ( 'NONE', ( #20192 ), #17703, .T. ) ;
#20327=EDGE_LOOP ( 'NONE', ( #6670, #12188, #15085, #13841 ) ) ;
#20330=EDGE_CURVE ( 'NONE', #12823, #1234, #23286, .T. ) ;
#20334=DIRECTION ( 'NONE',  ( -2.739037067331800130E-16, 0.000000000000000000, 1.000000000000000000 ) ) ;
#20352=ORIENTED_EDGE ( 'NONE', *, *, #357, .F. ) ;
#20354=CARTESIAN_POINT ( 'NONE',  ( -4.500000000000000000, -15.00000000000000000, -40.50000000000000000 ) ) ;
#20360=EDGE_LOOP ( 'NONE', ( #24491, #21962, #6821, #20418 ) ) ;
#20361=DIRECTION ( 'NONE',  ( 0.000000000000000000, 1.000000000000000000, 0.000000000000000000 ) ) ;
#20366=DIRECTION ( 'NONE',  ( -0.4151946956541399669, 0.5000000000001689759, -0.7600087925152558821 ) ) ;
#20371=DIRECTION ( 'NONE',  ( 0.000000000000000000, 1.000000000000000000, 0.000000000000000000 ) ) ;
#20377=ORIENTED_EDGE ( 'NONE', *, *, #7560, .F. ) ;
#20401=PRODUCT_DEFINITION_FORMATION_WITH_SPECIFIED_SOURCE ( 'ANY', '', #2252, .NOT_KNOWN. ) ;
#20418=ORIENTED_EDGE ( 'NONE', *, *, #3689, .F. ) ;
#20420=DIRECTION ( 'NONE',  ( 0.000000000000000000, 1.000000000000000000, 0.000000000000000000 ) ) ;
#20424=DIRECTION ( 'NONE',  ( 0.000000000000000000, 1.000000000000000000, 0.000000000000000000 ) ) ;
#20437=DIRECTION ( 'NONE',  ( 0.000000000000000000, 1.000000000000000000, 0.000000000000000000 ) ) ;
#20442=DIRECTION ( 'NONE',  ( 1.000000000000000000, 0.000000000000000000, 0.000000000000000000 ) ) ;
#20443=ADVANCED_FACE ( 'NONE', ( #19576 ), #12559, .F. ) ;
#20451=CARTESIAN_POINT ( 'NONE',  ( -40.50000000000000000, -15.00000000000000000, -4.500000000000000000 ) ) ;
#20457=CARTESIAN_POINT ( 'NONE',  ( 0.000000000000000000, -30.50310889129999836, 0.000000000000000000 ) ) ;
#20461=CARTESIAN_POINT ( 'NONE',  ( 0.000000000000000000, -39.50000000000000000, 0.000000000000000000 ) ) ;
#20475=AXIS2_PLACEMENT_3D ( 'NONE', #18375, #13992, #6859 ) ;
#20476=EDGE_CURVE ( 'NONE', #14401, #20122, #7498, .T. ) ;
#20479=EDGE_LOOP ( 'NONE', ( #12890, #7298, #22006, #9579 ) ) ;
#20484=CARTESIAN_POINT ( 'NONE',  ( 26.89647983300000078, -10.52212389379999991, 49.23367609159999603 ) ) ;
#20485=CARTESIAN_POINT ( 'NONE',  ( -5.873292863139999653, -11.55246854740000018, -10.75099047199999980 ) ) ;
#20505=DIRECTION ( 'NONE',  ( 0.4794255386042040601, 0.000000000000000000, 0.8775825618903720926 ) ) ;
#20519=ORIENTED_EDGE ( 'NONE', *, *, #20740, .F. ) ;
#20525=ORIENTED_EDGE ( 'NONE', *, *, #16181, .F. ) ;
#20526=DIRECTION ( 'NONE',  ( 0.4794255386042036715, 0.000000000000000000, 0.8775825618903723147 ) ) ;
#20536=CARTESIAN_POINT ( 'NONE',  ( -27.18988201479999844, -27.50155444569999830, -49.77074518290000071 ) ) ;
#20545=CIRCLE ( 'NONE', #9359, 57.75000000000000000 ) ;
#20546=UNCERTAINTY_MEASURE_WITH_UNIT (LENGTH_MEASURE( 1.000000000000000082E-05 ), #25669, 'distance_accuracy_value', 'NONE');
#20551=ORIENTED_EDGE ( 'NONE', *, *, #16680, .T. ) ;
#20553=VERTEX_POINT ( 'NONE', #21484 ) ;
#20557=DIRECTION ( 'NONE',  ( 0.4794255386042036715, 0.000000000000000000, 0.8775825618903724257 ) ) ;
#20568=CARTESIAN_POINT ( 'NONE',  ( 50.00000000000000000, -12.50000000000000000, -4.500000000000000000 ) ) ;
#20579=CARTESIAN_POINT ( 'NONE',  ( -26.77683864449999973, -30.20000000000000284, -49.01467436490000296 ) ) ;
#20589=DIRECTION ( 'NONE',  ( 0.4794255386042040601, 0.000000000000000000, 0.8775825618903720926 ) ) ;
#20608=DIRECTION ( 'NONE',  ( 1.000000000000000000, 0.000000000000000000, 0.000000000000000000 ) ) ;
#20612=DIRECTION ( 'NONE',  ( 0.4794255386042036160, 0.000000000000000000, 0.8775825618903723147 ) ) ;
#20621=ORIENTED_EDGE ( 'NONE', *, *, #19024, .F. ) ;
#20629=CARTESIAN_POINT ( 'NONE',  ( 0.000000000000000000, -2.000000000000000000, 0.000000000000000000 ) ) ;
#20631=CARTESIAN_POINT ( 'NONE',  ( 29.41275679339999982, -11.79999999999999893, 53.83969017199999740 ) ) ;
#20636=CARTESIAN_POINT ( 'NONE',  ( 27.68682485439999752, -24.80000000000000071, 50.68039294919999804 ) ) ;
#20652=VERTEX_POINT ( 'NONE', #20005 ) ;
#20654=FACE_OUTER_BOUND ( 'NONE', #28132, .T. ) ;
#20661=VERTEX_POINT ( 'NONE', #12397 ) ;
#20663=AXIS2_PLACEMENT_3D ( 'NONE', #21914, #1965, #20608 ) ;
#20687=DIRECTION ( 'NONE',  ( -0.4151946956541399669, 0.5000000000001689759, -0.7600087925152558821 ) ) ;
#20691=ORIENTED_EDGE ( 'NONE', *, *, #12897, .F. ) ;
#20697=ORIENTED_EDGE ( 'NONE', *, *, #7974, .T. ) ;
#20702=VECTOR ( 'NONE', #5208, 1000.000000000000000 ) ;
#20705=ORIENTED_EDGE ( 'NONE', *, *, #3911, .T. ) ;
#20727=CIRCLE ( 'NONE', #21195, 0.4999999999999981126 ) ;
#20739=VERTEX_POINT ( 'NONE', #12534 ) ;
#20740=EDGE_CURVE ( 'NONE', #1856, #15453, #1451, .T. ) ;
#20751=DIRECTION ( 'NONE',  ( 0.000000000000000000, 1.000000000000000000, 0.000000000000000000 ) ) ;
#20756=DIRECTION ( 'NONE',  ( 1.000000000000000000, 0.000000000000000000, 0.000000000000000000 ) ) ;
#20764=DIRECTION ( 'NONE',  ( -0.4151946956541399669, 0.5000000000001689759, -0.7600087925152558821 ) ) ;
#20765=AXIS2_PLACEMENT_3D ( 'NONE', #9619, #24935, #16474 ) ;
#20770=ORIENTED_EDGE ( 'NONE', *, *, #673, .F. ) ;
#20779=ADVANCED_FACE ( 'NONE', ( #4242 ), #6130, .T. ) ;
#20780=FACE_OUTER_BOUND ( 'NONE', #12567, .T. ) ;
#20782=EDGE_CURVE ( 'NONE', #17731, #20553, #16334, .T. ) ;
#20783=FACE_OUTER_BOUND ( 'NONE', #13561, .T. ) ;
#20794=CARTESIAN_POINT ( 'NONE',  ( 4.500000000000000000, -13.00000000000000000, 31.00000000000000000 ) ) ;
#20799=DIRECTION ( 'NONE',  ( 0.000000000000000000, 1.000000000000000000, 0.000000000000000000 ) ) ;
#20810=ADVANCED_FACE ( 'NONE', ( #8737 ), #19585, .T. ) ;
#20812=ORIENTED_EDGE ( 'NONE', *, *, #26009, .T. ) ;
#20820=ORIENTED_EDGE ( 'NONE', *, *, #27855, .T. ) ;
#20826=CARTESIAN_POINT ( 'NONE',  ( -27.18988201479999844, -18.49844555430000170, -49.77074518290000071 ) ) ;
#20828=AXIS2_PLACEMENT_3D ( 'NONE', #12375, #28393, #25937 ) ;
#20832=DIRECTION ( 'NONE',  ( 0.000000000000000000, 1.000000000000000000, 0.000000000000000000 ) ) ;
#20838=DIRECTION ( 'NONE',  ( 1.000000000000000000, 0.000000000000000000, 0.000000000000000000 ) ) ;
#20846=VERTEX_POINT ( 'NONE', #14005 ) ;
#20856=CIRCLE ( 'NONE', #1323, 57.75000000000000000 ) ;
#20862=VERTEX_POINT ( 'NONE', #23057 ) ;
#20866=CARTESIAN_POINT ( 'NONE',  ( 26.69293917519999937, -33.49689110869999809, 48.86109741659999628 ) ) ;
#20869=DIRECTION ( 'NONE',  ( 1.000000000000000000, 0.000000000000000000, 0.000000000000000000 ) ) ;
#20870=DIRECTION ( 'NONE',  ( 0.000000000000000000, 0.000000000000000000, 1.000000000000000000 ) ) ;
#20874=AXIS2_PLACEMENT_3D ( 'NONE', #28665, #12642, #25928 ) ;
#20876=DIRECTION ( 'NONE',  ( -0.8775825618903722036, 0.000000000000000000, 0.4794255386042041156 ) ) ;
#20893=DIRECTION ( 'NONE',  ( 0.4794255386042033384, 0.000000000000000000, 0.8775825618903726477 ) ) ;
#20895=VERTEX_POINT ( 'NONE', #20866 ) ;
#20923=FILL_AREA_STYLE ('',( #14220 ) ) ;
#20930=CIRCLE ( 'NONE', #8326, 55.67692378859999991 ) ;
#20931=VECTOR ( 'NONE', #14432, 1000.000000000000000 ) ;
#20945=ADVANCED_FACE ( 'NONE', ( #16179 ), #9767, .F. ) ;
#20956=ORIENTED_EDGE ( 'NONE', *, *, #2050, .F. ) ;
#20961=VERTEX_POINT ( 'NONE', #23471 ) ;
#20963=DIRECTION ( 'NONE',  ( -1.000000000000000000, 0.000000000000000000, 0.000000000000000000 ) ) ;
#20977=ORIENTED_EDGE ( 'NONE', *, *, #5630, .F. ) ;
#20982=ORIENTED_EDGE ( 'NONE', *, *, #13232, .T. ) ;
#20983=ADVANCED_FACE ( 'NONE', ( #7472 ), #25634, .F. ) ;
#20988=TOROIDAL_SURFACE ( 'NONE', #15842, 55.85192378860000417, 0.3499999999999999778 ) ;
#21000=DIRECTION ( 'NONE',  ( 0.4794255386042059475, 0.000000000000000000, 0.8775825618903710934 ) ) ;
#21015=CARTESIAN_POINT ( 'NONE',  ( -40.50000000000000000, -12.50000000000000000, -4.500000000000000000 ) ) ;
#21016=CIRCLE ( 'NONE', #4239, 57.75000000000000000 ) ;
#21020=AXIS2_PLACEMENT_3D ( 'NONE', #11432, #26908, #4757 ) ;
#21028=FACE_OUTER_BOUND ( 'NONE', #14976, .T. ) ;
#21030=FACE_OUTER_BOUND ( 'NONE', #22131, .T. ) ;
#21035=CIRCLE ( 'NONE', #7548, 24.50000000000000000 ) ;
#21038=DIRECTION ( 'NONE',  ( 1.000000000000000000, 0.000000000000000000, 0.000000000000000000 ) ) ;
#21053=EDGE_CURVE ( 'NONE', #9393, #26809, #12582, .T. ) ;
#21065=CARTESIAN_POINT ( 'NONE',  ( 29.41275679339999982, -25.00000000000000000, 53.83969017199999740 ) ) ;
#21067=EDGE_CURVE ( 'NONE', #13365, #20661, #20045, .T. ) ;
#21070=CARTESIAN_POINT ( 'NONE',  ( -5.753106463249999969, -2.000000000000000000, -10.53099074269999846 ) ) ;
#21072=ORIENTED_EDGE ( 'NONE', *, *, #25987, .F. ) ;
#21088=CARTESIAN_POINT ( 'NONE',  ( -4.500000000000000000, -15.00000000000000000, 50.00000000000000000 ) ) ;
#21099=ADVANCED_FACE ( 'NONE', ( #9841 ), #7072, .F. ) ;
#21127=LINE ( 'NONE', #14415, #1773 ) ;
#21142=ADVANCED_FACE ( 'NONE', ( #26151 ), #1048, .F. ) ;
#21151=ORIENTED_EDGE ( 'NONE', *, *, #27436, .T. ) ;
#21156=DIRECTION ( 'NONE',  ( 1.000000000000000000, 0.000000000000000000, 0.000000000000000000 ) ) ;
#21157=CARTESIAN_POINT ( 'NONE',  ( 0.000000000000000000, -19.09689110869999951, 0.000000000000000000 ) ) ;
#21175=EDGE_LOOP ( 'NONE', ( #24626, #19578, #8926, #9484 ) ) ;
#21176=ADVANCED_FACE ( 'NONE', ( #15480 ), #28320, .T. ) ;
#21195=AXIS2_PLACEMENT_3D ( 'NONE', #19801, #21854, #19943 ) ;
#21200=DIRECTION ( 'NONE',  ( 0.4794255386042000078, 0.000000000000000000, 0.8775825618903743131 ) ) ;
#21216=DIRECTION ( 'NONE',  ( 0.4794255386042041156, 0.000000000000000000, 0.8775825618903722036 ) ) ;
#21217=DIRECTION ( 'NONE',  ( 0.000000000000000000, 1.000000000000000000, 0.000000000000000000 ) ) ;
#21231=ADVANCED_FACE ( 'NONE', ( #15777 ), #22884, .T. ) ;
#21247=VERTEX_POINT ( 'NONE', #24832 ) ;
#21253=EDGE_CURVE ( 'NONE', #25637, #618, #9373, .T. ) ;
#21262=EDGE_LOOP ( 'NONE', ( #20691, #15418, #17361, #9923 ) ) ;
#21288=( NAMED_UNIT ( * ) PLANE_ANGLE_UNIT ( ) SI_UNIT ( $, .RADIAN. ) );
#21291=CIRCLE ( 'NONE', #3158, 0.3500000000000003664 ) ;
#21292=ADVANCED_FACE ( 'NONE', ( #21315 ), #25550, .T. ) ;
#21297=CARTESIAN_POINT ( 'NONE',  ( 0.000000000000000000, -15.80000000000000071, 0.000000000000000000 ) ) ;
#21308=LINE ( 'NONE', #18984, #11186 ) ;
#21315=FACE_OUTER_BOUND ( 'NONE', #24202, .T. ) ;
#21323=ORIENTED_EDGE ( 'NONE', *, *, #17105, .T. ) ;
#21328=CIRCLE ( 'NONE', #25064, 57.75000000000000000 ) ;
#21338=ORIENTED_EDGE ( 'NONE', *, *, #6311, .T. ) ;
#21345=DIRECTION ( 'NONE',  ( 0.4151946956541399669, 0.5000000000001689759, 0.7600087925152558821 ) ) ;
#21347=TOROIDAL_SURFACE ( 'NONE', #12478, 19.50000000000000000, 7.000000000000000000 ) ;
#21358=EDGE_CURVE ( 'NONE', #9863, #4043, #20066, .T. ) ;
#21364=CONICAL_SURFACE ( 'NONE', #9250, 8.099999999999997868, 0.7853981633970000820 ) ;
#21365=VECTOR ( 'NONE', #3707, 1000.000000000000114 ) ;
#21396=ORIENTED_EDGE ( 'NONE', *, *, #14417, .T. ) ;
#21406=AXIS2_PLACEMENT_3D ( 'NONE', #1843, #8105, #8524 ) ;
#21427=AXIS2_PLACEMENT_3D ( 'NONE', #14458, #23352, #28004 ) ;
#21430=ORIENTED_EDGE ( 'NONE', *, *, #28731, .T. ) ;
#21431=DIRECTION ( 'NONE',  ( 0.4794255386042040046, 0.000000000000000000, 0.8775825618903722036 ) ) ;
#21439=ORIENTED_EDGE ( 'NONE', *, *, #13655, .F. ) ;
#21440=DIRECTION ( 'NONE',  ( -0.8775825618903722036, 0.000000000000000000, 0.4794255386042041156 ) ) ;
#21445=AXIS2_PLACEMENT_3D ( 'NONE', #5219, #16273, #4923 ) ;
#21447=CARTESIAN_POINT ( 'NONE',  ( 25.77179612209999959, -37.57799544290000426, 47.17495636800000369 ) ) ;
#21448=VECTOR ( 'NONE', #22613, 1000.000000000000000 ) ;
#21451=DIRECTION ( 'NONE',  ( 0.000000000000000000, 1.000000000000000000, 0.000000000000000000 ) ) ;
#21452=ORIENTED_EDGE ( 'NONE', *, *, #5324, .T. ) ;
#21457=CARTESIAN_POINT ( 'NONE',  ( -27.68682485439999752, -13.40000000000000036, -50.68039294919999804 ) ) ;
#21459=DIRECTION ( 'NONE',  ( 0.4794255386042041156, 0.000000000000000000, 0.8775825618903722036 ) ) ;
#21472=DIRECTION ( 'NONE',  ( 1.000000000000000000, 0.000000000000000000, 0.000000000000000000 ) ) ;
#21475=CARTESIAN_POINT ( 'NONE',  ( 0.000000000000000000, -16.10310889129999623, 0.000000000000000000 ) ) ;
#21476=DIRECTION ( 'NONE',  ( 0.000000000000000000, 1.000000000000000000, 0.000000000000000000 ) ) ;
#21477=VERTEX_POINT ( 'NONE', #21457 ) ;
#21479=DIRECTION ( 'NONE',  ( 0.000000000000000000, 1.000000000000000000, 0.000000000000000000 ) ) ;
#21480=EDGE_LOOP ( 'NONE', ( #4629, #16256, #18909, #13216 ) ) ;
#21484=CARTESIAN_POINT ( 'NONE',  ( -6.831813925109999630, -13.50000000000000000, -12.50555150689999984 ) ) ;
#21488=AXIS2_PLACEMENT_3D ( 'NONE', #22916, #25247, #8019 ) ;
#21512=EDGE_CURVE ( 'NONE', #19954, #28714, #23780, .T. ) ;
#21517=PLANE ( 'NONE',  #6712 ) ;
#21520=VECTOR ( 'NONE', #7441, 1000.000000000000000 ) ;
#21521=CIRCLE ( 'NONE', #5255, 0.3500000000000003664 ) ;
#21532=VERTEX_POINT ( 'NONE', #24654 ) ;
#21533=VECTOR ( 'NONE', #703, 1000.000000000000000 ) ;
#21534=FACE_OUTER_BOUND ( 'NONE', #19240, .T. ) ;
#21542=ORIENTED_EDGE ( 'NONE', *, *, #3790, .T. ) ;
#21543=AXIS2_PLACEMENT_3D ( 'NONE', #25339, #14393, #3055 ) ;
#21550=CARTESIAN_POINT ( 'NONE',  ( 0.000000000000000000, -15.49689110870000164, 0.000000000000000000 ) ) ;
#21555=DIRECTION ( 'NONE',  ( 0.000000000000000000, 1.000000000000000000, 0.000000000000000000 ) ) ;
#21560=LINE ( 'NONE', #23601, #3804 ) ;
#21572=ORIENTED_EDGE ( 'NONE', *, *, #26209, .F. ) ;
#21576=ORIENTED_EDGE ( 'NONE', *, *, #5324, .F. ) ;
#21585=ORIENTED_EDGE ( 'NONE', *, *, #8902, .F. ) ;
#21598=AXIS2_PLACEMENT_3D ( 'NONE', #10610, #12670, #24044 ) ;
#21605=ORIENTED_EDGE ( 'NONE', *, *, #12276, .T. ) ;
#21626=DIRECTION ( 'NONE',  ( 0.4794255386042036715, 0.000000000000000000, 0.8775825618903723147 ) ) ;
#21630=DIRECTION ( 'NONE',  ( 0.4794255386042040046, 0.000000000000000000, 0.8775825618903722036 ) ) ;
#21651=CLOSED_SHELL ( 'NONE', ( #9812, #9036, #7730, #16433, #20443, #20983, #13241, #5216, #2085, #5346, #10744, #9007, #20316, #18378, #19317, #21832, #22757, #23085, #18401, #20810, #5930, #19849, #12034, #16149, #10428, #26188, #14118, #12480, #21231, #9828, #26241, #27571, #4010, #21176, #19647, #14359, #943, #22558, #7288, #14093, #23137, #28476, #28131, #13100, #24263, #27785, #19963, #21703, #14732, #12640, #11009, #28219, #24921, #28348, #8474, #22824, #467, #2992, #9706, #1840, #9617, #1134, #13746, #23815, #8963, #5481, #17290, #255, #16609, #2816, #19885, #19497, #14920, #11625, #368, #21142, #7792, #6754, #3027, #21099, #18274, #22447, #5351, #20171, #15305, #9859, #6013, #10242, #25774, #3253, #23749, #9347, #22992, #17631, #17890, #20945, #19532, #8097, #25767, #24009, #19399, #4817, #2240, #165, #2347, #16498, #10976, #17326, #20779, #15263, #21292, #1434, #6107, #25223, #16416, #8032, #5073, #28249, #13015, #27196, #20174, #14309, #17568, #6995, #22078, #125, #23942, #12381, #16999, #10000, #28409, #15100, #10623, #14542, #2457, #2154, #3878 ) ) ;
#21655=CARTESIAN_POINT ( 'NONE',  ( 2.220446049249999745E-14, -11.00000000000000000, -31.00000000000000000 ) ) ;
#21670=ORIENTED_EDGE ( 'NONE', *, *, #16751, .F. ) ;
#21671=EDGE_CURVE ( 'NONE', #8189, #584, #26843, .T. ) ;
#21697=EDGE_LOOP ( 'NONE', ( #11008, #2635, #16651, #20257 ) ) ;
#21698=CARTESIAN_POINT ( 'NONE',  ( 0.000000000000000000, -10.95575221240000019, 0.000000000000000000 ) ) ;
#21700=DIRECTION ( 'NONE',  ( 0.000000000000000000, 1.000000000000000000, 0.000000000000000000 ) ) ;
#21703=ADVANCED_FACE ( 'NONE', ( #18534 ), #26602, .F. ) ;
#21716=DIRECTION ( 'NONE',  ( 0.000000000000000000, 1.000000000000000000, 0.000000000000000000 ) ) ;
#21729=FACE_OUTER_BOUND ( 'NONE', #476, .T. ) ;
#21734=CIRCLE ( 'NONE', #13838, 12.00000000000000000 ) ;
#21746=AXIS2_PLACEMENT_3D ( 'NONE', #23479, #14845, #3927 ) ;
#21752=DIRECTION ( 'NONE',  ( 0.000000000000000000, -1.000000000000000000, 0.000000000000000000 ) ) ;
#21756=ORIENTED_EDGE ( 'NONE', *, *, #5630, .T. ) ;
#21763=EDGE_CURVE ( 'NONE', #3841, #2153, #18725, .T. ) ;
#21777=FACE_BOUND ( 'NONE', #9064, .T. ) ;
#21791=CIRCLE ( 'NONE', #28297, 57.75000000000000000 ) ;
#21793=CONICAL_SURFACE ( 'NONE', #24123, 21.60095686220001454, 0.7949521073230001456 ) ;
#21800=ORIENTED_EDGE ( 'NONE', *, *, #24795, .F. ) ;
#21806=ORIENTED_EDGE ( 'NONE', *, *, #12761, .F. ) ;
#21816=DIRECTION ( 'NONE',  ( 0.000000000000000000, 1.000000000000000000, 0.000000000000000000 ) ) ;
#21818=CARTESIAN_POINT ( 'NONE',  ( 27.68147801010000109, -38.34400911419999858, 50.67060561630000137 ) ) ;
#21821=ORIENTED_EDGE ( 'NONE', *, *, #11307, .T. ) ;
#21826=TOROIDAL_SURFACE ( 'NONE', #1834, 55.85192378860000417, 0.3499999999999999778 ) ;
#21832=ADVANCED_FACE ( 'NONE', ( #14009 ), #26149, .F. ) ;
#21833=CIRCLE ( 'NONE', #12064, 9.499999999999998224 ) ;
#21850=AXIS2_PLACEMENT_3D ( 'NONE', #13096, #17638, #28553 ) ;
#21851=CIRCLE ( 'NONE', #27923, 25.11294200180000047 ) ;
#21853=CARTESIAN_POINT ( 'NONE',  ( 0.000000000000000000, -19.09689110869999951, 0.000000000000000000 ) ) ;
#21854=DIRECTION ( 'NONE',  ( 0.8775825618903722036, 0.000000000000000000, -0.4794255386042041156 ) ) ;
#21876=EDGE_CURVE ( 'NONE', #7380, #4012, #21560, .T. ) ;
#21881=CIRCLE ( 'NONE', #26078, 57.75000000000000000 ) ;
#21887=DIRECTION ( 'NONE',  ( 1.000000000000000000, 0.000000000000000000, 0.000000000000000000 ) ) ;
#21903=ORIENTED_EDGE ( 'NONE', *, *, #13361, .T. ) ;
#21907=ORIENTED_EDGE ( 'NONE', *, *, #22826, .T. ) ;
#21914=CARTESIAN_POINT ( 'NONE',  ( -40.50000000000000000, -11.00000000000000000, 4.500000000000000000 ) ) ;
#21915=ORIENTED_EDGE ( 'NONE', *, *, #9637, .T. ) ;
#21920=CARTESIAN_POINT ( 'NONE',  ( 29.17304402409999753, -10.00000000000000000, 53.40089889099999709 ) ) ;
#21922=DIRECTION ( 'NONE',  ( 0.000000000000000000, 1.000000000000000000, 0.000000000000000000 ) ) ;
#21954=ORIENTED_EDGE ( 'NONE', *, *, #6518, .T. ) ;
#21962=ORIENTED_EDGE ( 'NONE', *, *, #27354, .T. ) ;
#21969=EDGE_LOOP ( 'NONE', ( #27371, #9262, #27473, #636 ) ) ;
#21982=ORIENTED_EDGE ( 'NONE', *, *, #19891, .F. ) ;
#21992=CARTESIAN_POINT ( 'NONE',  ( 0.000000000000000000, -11.50000000000000000, 0.000000000000000000 ) ) ;
#21997=CIRCLE ( 'NONE', #26120, 9.500000000000000000 ) ;
#22006=ORIENTED_EDGE ( 'NONE', *, *, #16884, .F. ) ;
#22016=AXIS2_PLACEMENT_3D ( 'NONE', #15017, #17227, #7790 ) ;
#22021=VERTEX_POINT ( 'NONE', #4801 ) ;
#22031=ORIENTED_EDGE ( 'NONE', *, *, #4275, .T. ) ;
#22044=ORIENTED_EDGE ( 'NONE', *, *, #5965, .T. ) ;
#22048=ORIENTED_EDGE ( 'NONE', *, *, #14459, .T. ) ;
#22056=DIRECTION ( 'NONE',  ( 0.8775825618903722036, 0.000000000000000000, -0.4794255386042041156 ) ) ;
#22065=CARTESIAN_POINT ( 'NONE',  ( -25.02601311510000315, -6.000000000000000000, -45.80980973070000317 ) ) ;
#22071=DIRECTION ( 'NONE',  ( 1.000000000000000000, 0.000000000000000000, 0.000000000000000000 ) ) ;
#22078=ADVANCED_FACE ( 'NONE', ( #10012, #16448 ), #27806, .F. ) ;
#22092=DIRECTION ( 'NONE',  ( 0.000000000000000000, 1.000000000000000000, 0.000000000000000000 ) ) ;
#22093=ORIENTED_EDGE ( 'NONE', *, *, #14502, .F. ) ;
#22104=CARTESIAN_POINT ( 'NONE',  ( -29.17304402409999753, -10.50000000000000000, -53.40089889099999709 ) ) ;
#22109=CARTESIAN_POINT ( 'NONE',  ( 0.000000000000000000, -23.30310889129999907, 0.000000000000000000 ) ) ;
#22130=CARTESIAN_POINT ( 'NONE',  ( 0.000000000000000000, -2.000000000000000000, 0.000000000000000000 ) ) ;
#22131=EDGE_LOOP ( 'NONE', ( #852, #25514, #12038, #7844 ) ) ;
#22134=FACE_OUTER_BOUND ( 'NONE', #12843, .T. ) ;
#22135=EDGE_CURVE ( 'NONE', #6364, #17271, #11705, .T. ) ;
#22147=AXIS2_PLACEMENT_3D ( 'NONE', #13456, #24536, #22071 ) ;
#22149=FACE_OUTER_BOUND ( 'NONE', #14052, .T. ) ;
#22160=DIRECTION ( 'NONE',  ( -1.186916062510446772E-15, 0.000000000000000000, 1.000000000000000000 ) ) ;
#22171=CARTESIAN_POINT ( 'NONE',  ( -4.123059632000000363, -17.00000000000000000, -7.547210032260000645 ) ) ;
#22174=ORIENTED_EDGE ( 'NONE', *, *, #669, .T. ) ;
#22178=DIRECTION ( 'NONE',  ( 1.000000000000000000, 0.000000000000000000, 0.000000000000000000 ) ) ;
#22186=FACE_OUTER_BOUND ( 'NONE', #18501, .T. ) ;
#22188=EDGE_LOOP ( 'NONE', ( #28401, #14323, #13769, #9636 ) ) ;
#22202=EDGE_LOOP ( 'NONE', ( #21915, #25687 ) ) ;
#22204=DIRECTION ( 'NONE',  ( 0.4794255386042000078, 0.000000000000000000, 0.8775825618903743131 ) ) ;
#22212=ORIENTED_EDGE ( 'NONE', *, *, #16593, .F. ) ;
#22226=ORIENTED_EDGE ( 'NONE', *, *, #6311, .F. ) ;
#22229=CARTESIAN_POINT ( 'NONE',  ( -12.03978574509999966, -15.00000000000000000, -22.03867997850000293 ) ) ;
#22245=EDGE_CURVE ( 'NONE', #519, #618, #24764, .T. ) ;
#22250=CARTESIAN_POINT ( 'NONE',  ( 0.000000000000000000, -39.32601556110000018, 0.000000000000000000 ) ) ;
#22255=AXIS2_PLACEMENT_3D ( 'NONE', #13227, #15854, #19786 ) ;
#22280=DIRECTION ( 'NONE',  ( 0.000000000000000000, 1.000000000000000000, 0.000000000000000000 ) ) ;
#22282=CIRCLE ( 'NONE', #26001, 0.9999999999999980016 ) ;
#22287=CARTESIAN_POINT ( 'NONE',  ( -26.69293917519999937, -26.90310889129999694, -48.86109741659999628 ) ) ;
#22289=EDGE_LOOP ( 'NONE', ( #7581, #2427, #1802, #14912 ) ) ;
#22291=CARTESIAN_POINT ( 'NONE',  ( 26.69293917519999937, -19.70310889130000120, 48.86109741659999628 ) ) ;
#22293=VECTOR ( 'NONE', #14739, 999.9999999999998863 ) ;
#22295=DIRECTION ( 'NONE',  ( 0.000000000000000000, 1.000000000000000000, 0.000000000000000000 ) ) ;
#22300=CIRCLE ( 'NONE', #28341, 61.35000000000000142 ) ;
#22314=DIRECTION ( 'NONE',  ( 0.000000000000000000, 1.000000000000000000, 0.000000000000000000 ) ) ;
#22322=CARTESIAN_POINT ( 'NONE',  ( 0.000000000000000000, -14.30000000000000071, 0.000000000000000000 ) ) ;
#22328=VERTEX_POINT ( 'NONE', #7035 ) ;
#22332=DIRECTION ( 'NONE',  ( 0.4794255386042041156, 0.000000000000000000, 0.8775825618903722036 ) ) ;
#22333=CARTESIAN_POINT ( 'NONE',  ( 0.000000000000000000, -28.10000000000000142, 0.000000000000000000 ) ) ;
#22334=VERTEX_POINT ( 'NONE', #18246 ) ;
#22354=DIRECTION ( 'NONE',  ( 0.000000000000000000, -1.000000000000000000, 0.000000000000000000 ) ) ;
#22357=FACE_OUTER_BOUND ( 'NONE', #11590, .T. ) ;
#22362=ORIENTED_EDGE ( 'NONE', *, *, #16459, .F. ) ;
#22363=DIRECTION ( 'NONE',  ( 1.000000000000000000, 0.000000000000000000, 0.000000000000000000 ) ) ;
#22402=DIRECTION ( 'NONE',  ( 0.4794255386042041156, 0.000000000000000000, 0.8775825618903720926 ) ) ;
#22410=EDGE_CURVE ( 'NONE', #13987, #14188, #16049, .T. ) ;
#22447=ADVANCED_FACE ( 'NONE', ( #9050 ), #4257, .T. ) ;
#22459=CARTESIAN_POINT ( 'NONE',  ( -25.57735248450000043, -16.00000000000000000, -46.81902967690000139 ) ) ;
#22466=DIRECTION ( 'NONE',  ( 0.000000000000000000, 1.000000000000000000, 0.000000000000000000 ) ) ;
#22475=VECTOR ( 'NONE', #24932, 1000.000000000000000 ) ;
#22480=CIRCLE ( 'NONE', #20133, 0.3500000000000003664 ) ;
#22484=FACE_OUTER_BOUND ( 'NONE', #28279, .T. ) ;
#22485=CARTESIAN_POINT ( 'NONE',  ( 0.000000000000000000, -10.95575221240000019, 0.000000000000000000 ) ) ;
#22495=EDGE_LOOP ( 'NONE', ( #5186, #16560, #23723, #18331 ) ) ;
#22509=DIRECTION ( 'NONE',  ( 0.000000000000000000, -1.000000000000000000, 0.000000000000000000 ) ) ;
#22512=CIRCLE ( 'NONE', #27170, 5.000000000000000000 ) ;
#22526=LINE ( 'NONE', #4591, #2260 ) ;
#22528=VECTOR ( 'NONE', #13376, 1000.000000000000000 ) ;
#22538=CARTESIAN_POINT ( 'NONE',  ( 0.000000000000000000, -10.50000000000000000, 0.000000000000000000 ) ) ;
#22547=FACE_OUTER_BOUND ( 'NONE', #19078, .T. ) ;
#22552=ORIENTED_EDGE ( 'NONE', *, *, #14543, .T. ) ;
#22558=ADVANCED_FACE ( 'NONE', ( #3796 ), #5679, .T. ) ;
#22563=VERTEX_POINT ( 'NONE', #17333 ) ;
#22567=CARTESIAN_POINT ( 'NONE',  ( 0.000000000000000000, -2.000000000000000000, 0.000000000000000000 ) ) ;
#22573=DIRECTION ( 'NONE',  ( 1.000000000000000000, 0.000000000000000000, 0.000000000000000000 ) ) ;
#22581=CARTESIAN_POINT ( 'NONE',  ( -27.68682485439999752, -17.89999999999999858, -50.68039294919999804 ) ) ;
#22604=LINE ( 'NONE', #25230, #9892 ) ;
#22613=DIRECTION ( 'NONE',  ( 0.000000000000000000, 1.000000000000000000, 0.000000000000000000 ) ) ;
#22614=DIRECTION ( 'NONE',  ( 0.4794255386042040046, 0.000000000000000000, 0.8775825618903722036 ) ) ;
#22619=CARTESIAN_POINT ( 'NONE',  ( 28.19022166989999789, -39.75000000000000000, 51.60185463919999194 ) ) ;
#22620=EDGE_CURVE ( 'NONE', #27211, #15688, #11727, .T. ) ;
#22631=CARTESIAN_POINT ( 'NONE',  ( 0.000000000000000000, -39.50000000000000000, 0.000000000000000000 ) ) ;
#22635=AXIS2_PLACEMENT_3D ( 'NONE', #7953, #9849, #5486 ) ;
#22644=EDGE_LOOP ( 'NONE', ( #22093, #1132, #10563, #16925 ) ) ;
#22671=ORIENTED_EDGE ( 'NONE', *, *, #8007, .T. ) ;
#22685=ORIENTED_EDGE ( 'NONE', *, *, #27498, .T. ) ;
#22695=AXIS2_PLACEMENT_3D ( 'NONE', #28123, #21700, #19509 ) ;
#22710=CARTESIAN_POINT ( 'NONE',  ( 26.69293917519999937, -16.10310889129999623, 48.86109741659999628 ) ) ;
#22728=ORIENTED_EDGE ( 'NONE', *, *, #2197, .F. ) ;
#22736=TOROIDAL_SURFACE ( 'NONE', #22255, 55.85192378860000417, 0.3499999999999999778 ) ;
#22742=ORIENTED_EDGE ( 'NONE', *, *, #28182, .T. ) ;
#22757=ADVANCED_FACE ( 'NONE', ( #2416 ), #20178, .T. ) ;
#22758=AXIS2_PLACEMENT_3D ( 'NONE', #7245, #5046, #18611 ) ;
#22765=CARTESIAN_POINT ( 'NONE',  ( 2.220446049249999745E-14, -11.00000000000000000, -50.00000000000000000 ) ) ;
#22770=CARTESIAN_POINT ( 'NONE',  ( 0.000000000000000000, -2.000000000000000000, 0.000000000000000000 ) ) ;
#22776=CIRCLE ( 'NONE', #9273, 52.35000000000000142 ) ;
#22795=AXIS2_PLACEMENT_3D ( 'NONE', #193, #6874, #15740 ) ;
#22815=DIRECTION ( 'NONE',  ( 0.4794255386042040046, 0.000000000000000000, 0.8775825618903722036 ) ) ;
#22817=CIRCLE ( 'NONE', #21406, 9.999999999999998224 ) ;
#22819=EDGE_CURVE ( 'NONE', #15502, #24319, #3289, .T. ) ;
#22820=ORIENTED_EDGE ( 'NONE', *, *, #12891, .F. ) ;
#22821=CARTESIAN_POINT ( 'NONE',  ( -28.07036528529999941, -39.32601556110000018, -51.38245899869999533 ) ) ;
#22823=ORIENTED_EDGE ( 'NONE', *, *, #5635, .T. ) ;
#22824=ADVANCED_FACE ( 'NONE', ( #25298 ), #27478, .T. ) ;
#22826=EDGE_CURVE ( 'NONE', #14525, #26731, #18276, .T. ) ;
#22829=DIRECTION ( 'NONE',  ( 0.8775825618903722036, 0.000000000000000000, -0.4794255386042041156 ) ) ;
#22838=CARTESIAN_POINT ( 'NONE',  ( 0.000000000000000000, -15.49689110870000164, 0.000000000000000000 ) ) ;
#22842=ORIENTED_EDGE ( 'NONE', *, *, #12208, .F. ) ;
#22844=AXIS2_PLACEMENT_3D ( 'NONE', #27687, #12344, #25628 ) ;
#22845=EDGE_CURVE ( 'NONE', #16409, #10454, #17318, .T. ) ;
#22854=DIRECTION ( 'NONE',  ( 0.4794255386042041156, 0.000000000000000000, 0.8775825618903720926 ) ) ;
#22862=CIRCLE ( 'NONE', #25195, 9.500000000000001776 ) ;
#22875=VERTEX_POINT ( 'NONE', #14485 ) ;
#22884=CONICAL_SURFACE ( 'NONE', #27051, 55.67692378859999280, 1.047197551199999799 ) ;
#22885=AXIS2_PLACEMENT_3D ( 'NONE', #15124, #8584, #12798 ) ;
#22904=DIRECTION ( 'NONE',  ( 1.000000000000000000, 0.000000000000000000, 0.000000000000000000 ) ) ;
#22909=AXIS2_PLACEMENT_3D ( 'NONE', #4655, #17626, #2487 ) ;
#22911=CARTESIAN_POINT ( 'NONE',  ( 0.000000000000000000, -24.50000000000000000, 0.000000000000000000 ) ) ;
#22915=FACE_OUTER_BOUND ( 'NONE', #20144, .T. ) ;
#22916=CARTESIAN_POINT ( 'NONE',  ( 0.000000000000000000, -19.40000000000000213, 0.000000000000000000 ) ) ;
#22928=EDGE_CURVE ( 'NONE', #28111, #9851, #9397, .T. ) ;
#22929=ORIENTED_EDGE ( 'NONE', *, *, #9377, .F. ) ;
#22938=PLANE ( 'NONE',  #23288 ) ;
#22942=ORIENTED_EDGE ( 'NONE', *, *, #18056, .T. ) ;
#22958=CARTESIAN_POINT ( 'NONE',  ( -29.17304402409999753, -10.00000000000000000, -53.40089889099999709 ) ) ;
#22969=DIRECTION ( 'NONE',  ( 0.4151946956541399669, 0.5000000000001689759, 0.7600087925152558821 ) ) ;
#22977=FACE_OUTER_BOUND ( 'NONE', #5942, .T. ) ;
#22984=DIRECTION ( 'NONE',  ( 0.4794255386042036715, 0.000000000000000000, 0.8775825618903724257 ) ) ;
#22992=ADVANCED_FACE ( 'NONE', ( #17816 ), #8928, .F. ) ;
#23010=DIRECTION ( 'NONE',  ( 0.4794255386042040601, 0.000000000000000000, 0.8775825618903720926 ) ) ;
#23013=CIRCLE ( 'NONE', #8098, 57.75000000000000000 ) ;
#23027=CARTESIAN_POINT ( 'NONE',  ( 0.000000000000000000, -39.50000000000000000, 0.000000000000000000 ) ) ;
#23028=VERTEX_POINT ( 'NONE', #2377 ) ;
#23034=CYLINDRICAL_SURFACE ( 'NONE', #9672, 57.74999999999999289 ) ;
#23035=ORIENTED_EDGE ( 'NONE', *, *, #18472, .T. ) ;
#23038=CONICAL_SURFACE ( 'NONE', #24876, 58.55000000000003979, 0.7853981633970000820 ) ;
#23050=CARTESIAN_POINT ( 'NONE',  ( 0.000000000000000000, -19.70310889130000120, 0.000000000000000000 ) ) ;
#23053=VERTEX_POINT ( 'NONE', #26557 ) ;
#23056=DIRECTION ( 'NONE',  ( 0.4794255386042041156, 0.000000000000000000, 0.8775825618903722036 ) ) ;
#23057=CARTESIAN_POINT ( 'NONE',  ( -27.68682485439999752, -28.10000000000000142, -50.68039294919999804 ) ) ;
#23059=CONICAL_SURFACE ( 'NONE', #28612, 55.67692378859999280, 1.047197551199999799 ) ;
#23060=DIRECTION ( 'NONE',  ( 0.000000000000000000, 1.000000000000000000, 0.000000000000000000 ) ) ;
#23074=DIRECTION ( 'NONE',  ( 0.000000000000000000, 1.000000000000000000, 0.000000000000000000 ) ) ;
#23075=ORIENTED_EDGE ( 'NONE', *, *, #2412, .T. ) ;
#23085=ADVANCED_FACE ( 'NONE', ( #22186 ), #2226, .T. ) ;
#23108=( NAMED_UNIT ( * ) SI_UNIT ( $, .STERADIAN. ) SOLID_ANGLE_UNIT ( ) );
#23110=DIRECTION ( 'NONE',  ( 1.000000000000000000, 0.000000000000000000, 0.000000000000000000 ) ) ;
#23125=DIRECTION ( 'NONE',  ( 0.4151946956541399669, 0.5000000000001689759, 0.7600087925152558821 ) ) ;
#23135=CARTESIAN_POINT ( 'NONE',  ( 31.00000000000000000, -15.00000000000000000, 2.042810365310000258E-14 ) ) ;
#23137=ADVANCED_FACE ( 'NONE', ( #8369 ), #8494, .F. ) ;
#23140=CARTESIAN_POINT ( 'NONE',  ( -27.18988201479999844, -31.10155444569999617, -49.77074518290000071 ) ) ;
#23142=ORIENTED_EDGE ( 'NONE', *, *, #26289, .F. ) ;
#23143=EDGE_CURVE ( 'NONE', #20652, #640, #26170, .T. ) ;
#23147=CARTESIAN_POINT ( 'NONE',  ( 0.000000000000000000, -39.32601556110000018, 0.000000000000000000 ) ) ;
#23149=TOROIDAL_SURFACE ( 'NONE', #367, 55.85192378860000417, 0.3499999999999999778 ) ;
#23163=CONICAL_SURFACE ( 'NONE', #10538, 55.67692378859999280, 1.047197551199999799 ) ;
#23176=ORIENTED_EDGE ( 'NONE', *, *, #8271, .F. ) ;
#23184=DIRECTION ( 'NONE',  ( 0.4794255386042040046, 0.000000000000000000, 0.8775825618903722036 ) ) ;
#23195=ORIENTED_EDGE ( 'NONE', *, *, #9705, .F. ) ;
#23206=ORIENTED_EDGE ( 'NONE', *, *, #2655, .T. ) ;
#23235=AXIS2_PLACEMENT_3D ( 'NONE', #21550, #10309, #23878 ) ;
#23247=SURFACE_STYLE_USAGE ( .BOTH. , #27634 ) ;
#23249=TOROIDAL_SURFACE ( 'NONE', #22795, 55.85192378860000417, 0.3499999999999999778 ) ;
#23267=ORIENTED_EDGE ( 'NONE', *, *, #456, .T. ) ;
#23271=AXIS2_PLACEMENT_3D ( 'NONE', #1494, #14314, #27596 ) ;
#23274=CARTESIAN_POINT ( 'NONE',  ( -4.500000000000000000, -11.00000000000000000, 50.00000000000000000 ) ) ;
#23275=EDGE_CURVE ( 'NONE', #14280, #3592, #12152, .T. ) ;
#23286=CIRCLE ( 'NONE', #14446, 57.73884739369999863 ) ;
#23288=AXIS2_PLACEMENT_3D ( 'NONE', #954, #27734, #1223 ) ;
#23302=EDGE_CURVE ( 'NONE', #23053, #11658, #19290, .T. ) ;
#23304=AXIS2_PLACEMENT_3D ( 'NONE', #18679, #7752, #16760 ) ;
#23306=CIRCLE ( 'NONE', #26561, 57.75000000000000000 ) ;
#23322=ORIENTED_EDGE ( 'NONE', *, *, #6748, .F. ) ;
#23340=DIRECTION ( 'NONE',  ( 0.000000000000000000, 1.000000000000000000, 0.000000000000000000 ) ) ;
#23347=ORIENTED_EDGE ( 'NONE', *, *, #25450, .T. ) ;
#23352=DIRECTION ( 'NONE',  ( 0.000000000000000000, 1.000000000000000000, 0.000000000000000000 ) ) ;
#23356=ORIENTED_EDGE ( 'NONE', *, *, #22410, .T. ) ;
#23373=AXIS2_PLACEMENT_3D ( 'NONE', #23571, #12754, #19617 ) ;
#23382=CARTESIAN_POINT ( 'NONE',  ( 0.000000000000000000, -2.000000000000000000, 0.000000000000000000 ) ) ;
#23391=CARTESIAN_POINT ( 'NONE',  ( -31.00000000000000000, -15.00000000000000000, -4.500000000000000000 ) ) ;
#23401=FACE_OUTER_BOUND ( 'NONE', #6126, .T. ) ;
#23406=EDGE_CURVE ( 'NONE', #23820, #3841, #22480, .T. ) ;
#23408=EDGE_LOOP ( 'NONE', ( #4910, #11799, #2087, #22226 ) ) ;
#23411=VECTOR ( 'NONE', #20366, 999.9999999999998863 ) ;
#23415=DIRECTION ( 'NONE',  ( 0.000000000000000000, 0.000000000000000000, 1.000000000000000000 ) ) ;
#23420=AXIS2_PLACEMENT_3D ( 'NONE', #15712, #463, #16013 ) ;
#23423=DIRECTION ( 'NONE',  ( -0.3422283636740854340, 0.7003189540771749266, -0.6264448177271558782 ) ) ;
#23442=ORIENTED_EDGE ( 'NONE', *, *, #19657, .T. ) ;
#23454=DIRECTION ( 'NONE',  ( 0.000000000000000000, 0.000000000000000000, -1.000000000000000000 ) ) ;
#23462=AXIS2_PLACEMENT_3D ( 'NONE', #1142, #3304, #7389 ) ;
#23467=VERTEX_POINT ( 'NONE', #18670 ) ;
#23471=CARTESIAN_POINT ( 'NONE',  ( -4.500000000000000000, -11.00000000000000000, -50.00000000000000000 ) ) ;
#23476=EDGE_LOOP ( 'NONE', ( #24959, #25838, #2609, #20551 ) ) ;
#23479=CARTESIAN_POINT ( 'NONE',  ( 0.000000000000000000, -19.70310889130000120, 0.000000000000000000 ) ) ;
#23521=DIRECTION ( 'NONE',  ( 0.000000000000000000, -1.000000000000000000, 0.000000000000000000 ) ) ;
#23529=DIRECTION ( 'NONE',  ( 0.4794255386042041711, 0.000000000000000000, 0.8775825618903720926 ) ) ;
#23552=CARTESIAN_POINT ( 'NONE',  ( -26.77683864449999973, -15.80000000000000071, -49.01467436490000296 ) ) ;
#23571=CARTESIAN_POINT ( 'NONE',  ( 9.348798002780000616, -10.50000000000000000, 17.11285995690000306 ) ) ;
#23572=ORIENTED_EDGE ( 'NONE', *, *, #1875, .T. ) ;
#23597=DIRECTION ( 'NONE',  ( 0.000000000000000000, 1.000000000000000000, 0.000000000000000000 ) ) ;
#23601=CARTESIAN_POINT ( 'NONE',  ( -27.18988201479999844, -32.89844555429999673, -49.77074518290000071 ) ) ;
#23604=DIRECTION ( 'NONE',  ( 0.8775825618903722036, 0.000000000000000000, -0.4794255386042041156 ) ) ;
#23607=LINE ( 'NONE', #3651, #13631 ) ;
#23608=AXIS2_PLACEMENT_3D ( 'NONE', #8845, #17609, #4349 ) ;
#23610=EDGE_CURVE ( 'NONE', #28111, #8881, #15452, .T. ) ;
#23611=AXIS2_PLACEMENT_3D ( 'NONE', #14575, #26225, #10321 ) ;
#23614=DIRECTION ( 'NONE',  ( -0.4151946956541399669, 0.5000000000001689759, -0.7600087925152558821 ) ) ;
#23618=PLANE ( 'NONE',  #23271 ) ;
#23635=EDGE_LOOP ( 'NONE', ( #18867, #550, #8210, #1170 ) ) ;
#23652=CIRCLE ( 'NONE', #19005, 53.35000000000000142 ) ;
#23659=EDGE_CURVE ( 'NONE', #22021, #2012, #6680, .T. ) ;
#23661=DIRECTION ( 'NONE',  ( 0.000000000000000000, 1.000000000000000000, 0.000000000000000000 ) ) ;
#23671=CIRCLE ( 'NONE', #22758, 9.499999999999998224 ) ;
#23672=CARTESIAN_POINT ( 'NONE',  ( 0.000000000000000000, -17.30000000000000071, 0.000000000000000000 ) ) ;
#23681=DIRECTION ( 'NONE',  ( 0.4794255386042036715, 0.000000000000000000, 0.8775825618903724257 ) ) ;
#23709=AXIS2_PLACEMENT_3D ( 'NONE', #23552, #25604, #27787 ) ;
#23717=DIRECTION ( 'NONE',  ( 0.4794255386042036715, 0.000000000000000000, 0.8775825618903724257 ) ) ;
#23720=ORIENTED_EDGE ( 'NONE', *, *, #673, .T. ) ;
#23723=ORIENTED_EDGE ( 'NONE', *, *, #17670, .T. ) ;
#23731=CIRCLE ( 'NONE', #14875, 12.25068835559999947 ) ;
#23745=DIRECTION ( 'NONE',  ( 0.000000000000000000, 1.000000000000000000, 0.000000000000000000 ) ) ;
#23749=ADVANCED_FACE ( 'NONE', ( #27525 ), #9435, .F. ) ;
#23751=AXIS2_PLACEMENT_3D ( 'NONE', #14902, #8772, #12715 ) ;
#23753=AXIS2_PLACEMENT_3D ( 'NONE', #26921, #11144, #24735 ) ;
#23763=FACE_BOUND ( 'NONE', #27597, .T. ) ;
#23770=DIRECTION ( 'NONE',  ( -0.8775825618903722036, 0.000000000000000000, 0.4794255386042041156 ) ) ;
#23774=ORIENTED_EDGE ( 'NONE', *, *, #5385, .T. ) ;
#23776=CIRCLE ( 'NONE', #11190, 53.75557630320000868 ) ;
#23780=LINE ( 'NONE', #26261, #23796 ) ;
#23783=FACE_OUTER_BOUND ( 'NONE', #1536, .T. ) ;
#23785=CARTESIAN_POINT ( 'NONE',  ( 26.77683864449999973, -33.79999999999999716, 49.01467436490000296 ) ) ;
#23788=EDGE_CURVE ( 'NONE', #15502, #25637, #9719, .T. ) ;
#23796=VECTOR ( 'NONE', #28284, 1000.000000000000000 ) ;
#23797=CIRCLE ( 'NONE', #27054, 9.500000000000001776 ) ;
#23806=ORIENTED_EDGE ( 'NONE', *, *, #20137, .F. ) ;
#23812=FACE_OUTER_BOUND ( 'NONE', #2907, .T. ) ;
#23815=ADVANCED_FACE ( 'NONE', ( #18338 ), #19215, .F. ) ;
#23820=VERTEX_POINT ( 'NONE', #22710 ) ;
#23835=DIRECTION ( 'NONE',  ( 0.8775825618903722036, 0.000000000000000000, -0.4794255386042041156 ) ) ;
#23857=AXIS2_PLACEMENT_3D ( 'NONE', #18834, #28125, #27723 ) ;
#23861=ORIENTED_EDGE ( 'NONE', *, *, #17570, .F. ) ;
#23872=FACE_BOUND ( 'NONE', #16787, .T. ) ;
#23874=ORIENTED_EDGE ( 'NONE', *, *, #15531, .T. ) ;
#23878=DIRECTION ( 'NONE',  ( 1.000000000000000000, 0.000000000000000000, 0.000000000000000000 ) ) ;
#23883=DIRECTION ( 'NONE',  ( 0.000000000000000000, 1.000000000000000000, 0.000000000000000000 ) ) ;
#23898=EDGE_CURVE ( 'NONE', #87, #11019, #12682, .T. ) ;
#23901=CIRCLE ( 'NONE', #207, 0.3500000000000003664 ) ;
#23942=ADVANCED_FACE ( 'NONE', ( #14035 ), #25739, .F. ) ;
#23944=DIRECTION ( 'NONE',  ( 1.000000000000000000, 0.000000000000000000, 0.000000000000000000 ) ) ;
#23950=ORIENTED_EDGE ( 'NONE', *, *, #7161, .F. ) ;
#23966=ORIENTED_EDGE ( 'NONE', *, *, #20297, .T. ) ;
#23973=EDGE_CURVE ( 'NONE', #11658, #14011, #25753, .T. ) ;
#23988=VERTEX_POINT ( 'NONE', #25685 ) ;
#24009=ADVANCED_FACE ( 'NONE', ( #9934 ), #14320, .F. ) ;
#24013=ORIENTED_EDGE ( 'NONE', *, *, #13655, .T. ) ;
#24017=ORIENTED_EDGE ( 'NONE', *, *, #2629, .T. ) ;
#24026=LINE ( 'NONE', #10735, #22528 ) ;
#24044=DIRECTION ( 'NONE',  ( 0.4794255386042040601, 0.000000000000000000, 0.8775825618903720926 ) ) ;
#24045=DIRECTION ( 'NONE',  ( 0.4794255386042041711, 0.000000000000000000, 0.8775825618903720926 ) ) ;
#24052=DIRECTION ( 'NONE',  ( -1.836909530729999990E-16, 0.000000000000000000, 1.000000000000000000 ) ) ;
#24065=CARTESIAN_POINT ( 'NONE',  ( 26.60903970598167589, -23.00000000000000000, 48.70752046822583736 ) ) ;
#24066=DIRECTION ( 'NONE',  ( 1.000000000000000000, 0.000000000000000000, 0.000000000000000000 ) ) ;
#24072=EDGE_CURVE ( 'NONE', #258, #11126, #26206, .T. ) ;
#24095=CARTESIAN_POINT ( 'NONE',  ( 0.000000000000000000, -2.000000000000000000, 0.000000000000000000 ) ) ;
#24102=DIRECTION ( 'NONE',  ( -0.4151946956541399669, 0.5000000000001689759, -0.7600087925152558821 ) ) ;
#24105=EDGE_LOOP ( 'NONE', ( #6954, #15407, #12441, #12053 ) ) ;
#24123=AXIS2_PLACEMENT_3D ( 'NONE', #16578, #18779, #4928 ) ;
#24140=FACE_OUTER_BOUND ( 'NONE', #3199, .T. ) ;
#24146=VECTOR ( 'NONE', #17990, 1000.000000000000000 ) ;
#24164=CIRCLE ( 'NONE', #19514, 57.75000000000000000 ) ;
#24166=DIRECTION ( 'NONE',  ( 0.000000000000000000, 1.000000000000000000, 0.000000000000000000 ) ) ;
#24168=DIRECTION ( 'NONE',  ( 1.000000000000000000, 0.000000000000000000, 0.000000000000000000 ) ) ;
#24173=ORIENTED_EDGE ( 'NONE', *, *, #11591, .T. ) ;
#24178=DIRECTION ( 'NONE',  ( 0.000000000000000000, 1.000000000000000000, 0.000000000000000000 ) ) ;
#24183=TOROIDAL_SURFACE ( 'NONE', #4659, 55.85192378860000417, 0.3499999999999999778 ) ;
#24184=TOROIDAL_SURFACE ( 'NONE', #19515, 53.85000000000000142, 0.5000000000000000000 ) ;
#24186=DIRECTION ( 'NONE',  ( 0.000000000000000000, 1.000000000000000000, 0.000000000000000000 ) ) ;
#24202=EDGE_LOOP ( 'NONE', ( #20820, #23356, #22820, #20956 ) ) ;
#24205=DIRECTION ( 'NONE',  ( 0.000000000000000000, 1.000000000000000000, 0.000000000000000000 ) ) ;
#24211=ORIENTED_EDGE ( 'NONE', *, *, #1381, .F. ) ;
#24215=AXIS2_PLACEMENT_3D ( 'NONE', #3685, #19548, #21887 ) ;
#24233=CARTESIAN_POINT ( 'NONE',  ( 0.000000000000000000, -17.50000000000000000, 0.000000000000000000 ) ) ;
#24235=ORIENTED_EDGE ( 'NONE', *, *, #18904, .F. ) ;
#24247=DIRECTION ( 'NONE',  ( 0.000000000000000000, 1.000000000000000000, 0.000000000000000000 ) ) ;
#24263=ADVANCED_FACE ( 'NONE', ( #25378 ), #11791, .T. ) ;
#24268=AXIS2_PLACEMENT_3D ( 'NONE', #3106, #11958, #10179 ) ;
#24270=AXIS2_PLACEMENT_3D ( 'NONE', #16772, #5694, #1752 ) ;
#24280=DIRECTION ( 'NONE',  ( 0.4794255386042033384, 0.000000000000000000, 0.8775825618903726477 ) ) ;
#24286=CARTESIAN_POINT ( 'NONE',  ( 0.000000000000000000, -26.29689110869999880, 0.000000000000000000 ) ) ;
#24296=FACE_OUTER_BOUND ( 'NONE', #12773, .T. ) ;
#24299=CARTESIAN_POINT ( 'NONE',  ( 11.74592569580000045, -11.00000000000000000, 21.50077276629999901 ) ) ;
#24301=EDGE_CURVE ( 'NONE', #11029, #18513, #5762, .T. ) ;
#24314=DIRECTION ( 'NONE',  ( 0.4794255386042040601, 0.000000000000000000, 0.8775825618903720926 ) ) ;
#24316=DIRECTION ( 'NONE',  ( 1.000000000000000000, 0.000000000000000000, 0.000000000000000000 ) ) ;
#24319=VERTEX_POINT ( 'NONE', #16475 ) ;
#24340=ORIENTED_EDGE ( 'NONE', *, *, #5013, .F. ) ;
#24342=AXIS2_PLACEMENT_3D ( 'NONE', #7036, #11520, #27288 ) ;
#24355=LINE ( 'NONE', #22171, #18802 ) ;
#24371=ORIENTED_EDGE ( 'NONE', *, *, #22135, .F. ) ;
#24374=DIRECTION ( 'NONE',  ( 0.000000000000000000, -1.000000000000000000, 0.000000000000000000 ) ) ;
#24386=AXIS2_PLACEMENT_3D ( 'NONE', #25007, #7689, #16554 ) ;
#24400=VERTEX_POINT ( 'NONE', #27971 ) ;
#24407=AXIS2_PLACEMENT_3D ( 'NONE', #25824, #21440, #1768 ) ;
#24413=DIRECTION ( 'NONE',  ( 0.4794255386042000078, 0.000000000000000000, 0.8775825618903743131 ) ) ;
#24418=DIRECTION ( 'NONE',  ( 0.4794255386042040601, 0.000000000000000000, 0.8775825618903720926 ) ) ;
#24419=TOROIDAL_SURFACE ( 'NONE', #10901, 52.20000000000000284, 5.000000000000000000 ) ;
#24438=DIRECTION ( 'NONE',  ( 1.000000000000000000, 0.000000000000000000, 0.000000000000000000 ) ) ;
#24459=DIRECTION ( 'NONE',  ( 0.000000000000000000, 1.000000000000000000, 0.000000000000000000 ) ) ;
#24465=LINE ( 'NONE', #8, #2052 ) ;
#24468=DIRECTION ( 'NONE',  ( 1.000000000000000000, 0.000000000000000000, 0.000000000000000000 ) ) ;
#24480=ORIENTED_EDGE ( 'NONE', *, *, #11404, .F. ) ;
#24485=ORIENTED_EDGE ( 'NONE', *, *, #9159, .F. ) ;
#24491=ORIENTED_EDGE ( 'NONE', *, *, #13361, .F. ) ;
#24496=ORIENTED_EDGE ( 'NONE', *, *, #13517, .F. ) ;
#24508=CARTESIAN_POINT ( 'NONE',  ( 0.000000000000000000, -15.14308496720000008, 0.000000000000000000 ) ) ;
#24530=CIRCLE ( 'NONE', #17559, 55.67692378859999991 ) ;
#24536=DIRECTION ( 'NONE',  ( 0.000000000000000000, 1.000000000000000000, 0.000000000000000000 ) ) ;
#24541=CARTESIAN_POINT ( 'NONE',  ( 0.000000000000000000, -15.00000000000000000, 0.000000000000000000 ) ) ;
#24560=FACE_OUTER_BOUND ( 'NONE', #12266, .T. ) ;
#24565=AXIS2_PLACEMENT_3D ( 'NONE', #14062, #18297, #22815 ) ;
#24570=AXIS2_PLACEMENT_3D ( 'NONE', #9910, #16759, #23056 ) ;
#24588=VECTOR ( 'NONE', #26806, 1000.000000000000000 ) ;
#24592=CARTESIAN_POINT ( 'NONE',  ( -40.50000000000000000, -12.50000000000000000, 4.500000000000000000 ) ) ;
#24594=CARTESIAN_POINT ( 'NONE',  ( 27.68682485439999752, -13.40000000000000036, 50.68039294919999804 ) ) ;
#24603=CYLINDRICAL_SURFACE ( 'NONE', #17643, 57.74999999999999289 ) ;
#24626=ORIENTED_EDGE ( 'NONE', *, *, #23788, .F. ) ;
#24634=VECTOR ( 'NONE', #9175, 1000.000000000000000 ) ;
#24646=DIRECTION ( 'NONE',  ( 1.000000000000000000, 0.000000000000000000, 0.000000000000000000 ) ) ;
#24647=LINE ( 'NONE', #20568, #21448 ) ;
#24652=CARTESIAN_POINT ( 'NONE',  ( 0.000000000000000000, -13.40000000000000036, 0.000000000000000000 ) ) ;
#24654=CARTESIAN_POINT ( 'NONE',  ( 12.03978574509999966, -15.00000000000000000, 22.03867997850000293 ) ) ;
#24660=VECTOR ( 'NONE', #15025, 1000.000000000000114 ) ;
#24680=EDGE_CURVE ( 'NONE', #15502, #19846, #27179, .T. ) ;
#24689=CARTESIAN_POINT ( 'NONE',  ( 25.57735248450000043, -37.08699221940000257, 46.81902967690000139 ) ) ;
#24692=CARTESIAN_POINT ( 'NONE',  ( 29.08514934200000113, -10.00000000000000000, 53.24000875469999983 ) ) ;
#24698=CIRCLE ( 'NONE', #20021, 19.50000000000000000 ) ;
#24700=AXIS2_PLACEMENT_3D ( 'NONE', #24286, #26040, #13202 ) ;
#24716=CARTESIAN_POINT ( 'NONE',  ( -3.883346862689999845, -2.000000000000000000, -7.108418751309999450 ) ) ;
#24719=AXIS2_PLACEMENT_3D ( 'NONE', #15003, #12817, #24052 ) ;
#24720=FACE_BOUND ( 'NONE', #22495, .T. ) ;
#24724=AXIS2_PLACEMENT_3D ( 'NONE', #15938, #24845, #9233 ) ;
#24735=DIRECTION ( 'NONE',  ( 1.000000000000000000, 0.000000000000000000, 0.000000000000000000 ) ) ;
#24742=AXIS2_PLACEMENT_3D ( 'NONE', #6820, #15981, #13058 ) ;
#24749=ORIENTED_EDGE ( 'NONE', *, *, #12507, .F. ) ;
#24762=CARTESIAN_POINT ( 'NONE',  ( -29.41275679339999982, -39.50000000000000000, -53.83969017199999740 ) ) ;
#24763=LINE ( 'NONE', #17913, #24588 ) ;
#24764=CIRCLE ( 'NONE', #16378, 9.500000000000000000 ) ;
#24767=EDGE_LOOP ( 'NONE', ( #3022, #3185 ) ) ;
#24768=DIRECTION ( 'NONE',  ( -1.000000000000000000, 0.000000000000000000, 0.000000000000000000 ) ) ;
#24779=AXIS2_PLACEMENT_3D ( 'NONE', #8595, #5612, #12014 ) ;
#24795=EDGE_CURVE ( 'NONE', #22, #21247, #24355, .T. ) ;
#24801=CARTESIAN_POINT ( 'NONE',  ( 0.000000000000000000, -30.20000000000000284, 0.000000000000000000 ) ) ;
#24832=CARTESIAN_POINT ( 'NONE',  ( -3.883346862689999845, -16.50000000000000000, -7.108418751309999450 ) ) ;
#24845=DIRECTION ( 'NONE',  ( 0.000000000000000000, 1.000000000000000000, 0.000000000000000000 ) ) ;
#24848=EDGE_CURVE ( 'NONE', #19645, #8365, #1930, .T. ) ;
#24855=CIRCLE ( 'NONE', #17859, 57.75000000000000000 ) ;
#24862=DIRECTION ( 'NONE',  ( -0.8775825618903722036, 0.000000000000000000, 0.4794255386042041156 ) ) ;
#24876=AXIS2_PLACEMENT_3D ( 'NONE', #12713, #25994, #21626 ) ;
#24883=AXIS2_PLACEMENT_3D ( 'NONE', #26583, #20167, #84 ) ;
#24889=DIRECTION ( 'NONE',  ( 1.000000000000000000, 0.000000000000000000, 0.000000000000000000 ) ) ;
#24901=ORIENTED_EDGE ( 'NONE', *, *, #10114, .F. ) ;
#24904=DIRECTION ( 'NONE',  ( 1.000000000000000000, 0.000000000000000000, 0.000000000000000000 ) ) ;
#24912=VECTOR ( 'NONE', #19353, 999.9999999999998863 ) ;
#24918=ORIENTED_EDGE ( 'NONE', *, *, #17270, .T. ) ;
#24921=ADVANCED_FACE ( 'NONE', ( #4837 ), #15987, .T. ) ;
#24925=EDGE_CURVE ( 'NONE', #21477, #4628, #28544, .T. ) ;
#24927=CARTESIAN_POINT ( 'NONE',  ( -29.17304402409999753, -40.00000000000000000, -53.40089889099999709 ) ) ;
#24932=DIRECTION ( 'NONE',  ( 0.000000000000000000, 1.000000000000000000, 0.000000000000000000 ) ) ;
#24935=DIRECTION ( 'NONE',  ( 0.000000000000000000, 1.000000000000000000, 0.000000000000000000 ) ) ;
#24939=ORIENTED_EDGE ( 'NONE', *, *, #16186, .T. ) ;
#24950=DIRECTION ( 'NONE',  ( -0.8775825618903722036, 0.000000000000000000, 0.4794255386042041156 ) ) ;
#24951=CARTESIAN_POINT ( 'NONE',  ( -31.00000000000000000, -13.00000000000000000, 4.500000000000000000 ) ) ;
#24959=ORIENTED_EDGE ( 'NONE', *, *, #11749, .T. ) ;
#24962=CARTESIAN_POINT ( 'NONE',  ( 0.000000000000000000, -10.08849557519999962, 0.000000000000000000 ) ) ;
#24998=ORIENTED_EDGE ( 'NONE', *, *, #23143, .F. ) ;
#25000=DIRECTION ( 'NONE',  ( 0.000000000000000000, 1.000000000000000000, 0.000000000000000000 ) ) ;
#25007=CARTESIAN_POINT ( 'NONE',  ( 4.500000000000000000, 0.000000000000000000, 50.00000000000000000 ) ) ;
#25032=CARTESIAN_POINT ( 'NONE',  ( -26.77683864449999973, -30.20000000000000284, -49.01467436490000296 ) ) ;
#25037=DIRECTION ( 'NONE',  ( 0.000000000000000000, 1.000000000000000000, 0.000000000000000000 ) ) ;
#25041=EDGE_LOOP ( 'NONE', ( #26521, #26171, #11370, #15456 ) ) ;
#25043=FACE_OUTER_BOUND ( 'NONE', #14777, .T. ) ;
#25060=DIRECTION ( 'NONE',  ( 0.000000000000000000, 1.000000000000000000, 0.000000000000000000 ) ) ;
#25064=AXIS2_PLACEMENT_3D ( 'NONE', #19192, #1441, #8117 ) ;
#25093=CARTESIAN_POINT ( 'NONE',  ( -29.41275679339999982, -10.50000000000000000, -53.83969017199999740 ) ) ;
#25095=ORIENTED_EDGE ( 'NONE', *, *, #22410, .F. ) ;
#25097=CARTESIAN_POINT ( 'NONE',  ( 9.348798002780000616, -17.50000000000000000, 17.11285995690000306 ) ) ;
#25106=CIRCLE ( 'NONE', #1819, 57.75000000000000000 ) ;
#25107=AXIS2_PLACEMENT_3D ( 'NONE', #6127, #26252, #8047 ) ;
#25109=DIRECTION ( 'NONE',  ( 0.000000000000000000, 1.000000000000000000, 0.000000000000000000 ) ) ;
#25110=AXIS2_PLACEMENT_3D ( 'NONE', #8310, #24205, #4391 ) ;
#25116=CARTESIAN_POINT ( 'NONE',  ( 0.000000000000000000, -15.80000000000000071, 0.000000000000000000 ) ) ;
#25123=DIRECTION ( 'NONE',  ( 0.000000000000000000, 1.000000000000000000, 0.000000000000000000 ) ) ;
#25127=TOROIDAL_SURFACE ( 'NONE', #1394, 60.85000000000000142, 0.5000000000000000000 ) ;
#25133=CIRCLE ( 'NONE', #3276, 59.33923303830000151 ) ;
#25149=AXIS2_PLACEMENT_3D ( 'NONE', #6116, #2194, #28405 ) ;
#25154=CARTESIAN_POINT ( 'NONE',  ( 27.68682485439999752, -31.69999999999999929, 50.68039294919999804 ) ) ;
#25155=VERTEX_POINT ( 'NONE', #10316 ) ;
#25156=CARTESIAN_POINT ( 'NONE',  ( -25.09792694589999940, -15.00000000000000000, -45.94144711499999545 ) ) ;
#25159=DIRECTION ( 'NONE',  ( 0.4794255386042041156, 0.000000000000000000, 0.8775825618903720926 ) ) ;
#25175=TOROIDAL_SURFACE ( 'NONE', #7032, 55.85192378860000417, 0.3499999999999999778 ) ;
#25189=ORIENTED_EDGE ( 'NONE', *, *, #352, .F. ) ;
#25195=AXIS2_PLACEMENT_3D ( 'NONE', #20451, #4714, #20756 ) ;
#25199=EDGE_LOOP ( 'NONE', ( #11248, #27691, #21542, #18829 ) ) ;
#25215=VECTOR ( 'NONE', #2783, 1000.000000000000000 ) ;
#25218=EDGE_CURVE ( 'NONE', #12823, #14426, #8421, .T. ) ;
#25223=ADVANCED_FACE ( 'NONE', ( #17616 ), #704, .F. ) ;
#25230=CARTESIAN_POINT ( 'NONE',  ( -31.00000000000000000, -13.00000000000000000, -4.500000000000000000 ) ) ;
#25240=CARTESIAN_POINT ( 'NONE',  ( -50.00000000000000000, -11.00000000000000000, -2.486899575159999765E-14 ) ) ;
#25243=DIRECTION ( 'NONE',  ( 0.000000000000000000, 1.000000000000000000, 0.000000000000000000 ) ) ;
#25247=DIRECTION ( 'NONE',  ( 0.000000000000000000, 1.000000000000000000, 0.000000000000000000 ) ) ;
#25255=DIRECTION ( 'NONE',  ( 1.000000000000000000, 0.000000000000000000, 0.000000000000000000 ) ) ;
#25257=AXIS2_PLACEMENT_3D ( 'NONE', #23382, #14348, #1252 ) ;
#25268=FACE_BOUND ( 'NONE', #18623, .T. ) ;
#25280=AXIS2_PLACEMENT_3D ( 'NONE', #8590, #11037, #17933 ) ;
#25282=VECTOR ( 'NONE', #21752, 1000.000000000000000 ) ;
#25285=DIRECTION ( 'NONE',  ( 1.000000000000000000, 0.000000000000000000, 0.000000000000000000 ) ) ;
#25298=FACE_OUTER_BOUND ( 'NONE', #16115, .T. ) ;
#25305=ORIENTED_EDGE ( 'NONE', *, *, #24848, .T. ) ;
#25308=ORIENTED_EDGE ( 'NONE', *, *, #5155, .T. ) ;
#25323=CARTESIAN_POINT ( 'NONE',  ( -27.18988201479999844, -20.30155444569999901, -49.77074518290000071 ) ) ;
#25336=ORIENTED_EDGE ( 'NONE', *, *, #8666, .F. ) ;
#25338=CARTESIAN_POINT ( 'NONE',  ( -4.500000000000000000, 0.000000000000000000, -50.00000000000000000 ) ) ;
#25339=CARTESIAN_POINT ( 'NONE',  ( 0.000000000000000000, -16.00000000000000000, 0.000000000000000000 ) ) ;
#25340=CARTESIAN_POINT ( 'NONE',  ( 0.000000000000000000, -11.85850980319999870, 0.000000000000000000 ) ) ;
#25369=LINE ( 'NONE', #11795, #11383 ) ;
#25370=ORIENTED_EDGE ( 'NONE', *, *, #26696, .F. ) ;
#25375=DIRECTION ( 'NONE',  ( 0.000000000000000000, 1.000000000000000000, 0.000000000000000000 ) ) ;
#25378=FACE_OUTER_BOUND ( 'NONE', #2775, .T. ) ;
#25409=ORIENTED_EDGE ( 'NONE', *, *, #19619, .F. ) ;
#25417=LINE ( 'NONE', #18277, #28785 ) ;
#25450=EDGE_CURVE ( 'NONE', #8830, #28301, #14160, .T. ) ;
#25464=ORIENTED_EDGE ( 'NONE', *, *, #14417, .F. ) ;
#25487=AXIS2_PLACEMENT_3D ( 'NONE', #9342, #20424, #27285 ) ;
#25494=ORIENTED_EDGE ( 'NONE', *, *, #11467, .F. ) ;
#25503=FACE_OUTER_BOUND ( 'NONE', #2718, .T. ) ;
#25511=CARTESIAN_POINT ( 'NONE',  ( -11.87191034930000022, -15.14308496720000008, -21.73138612759999688 ) ) ;
#25514=ORIENTED_EDGE ( 'NONE', *, *, #12389, .T. ) ;
#25525=ADVANCED_BREP_SHAPE_REPRESENTATION ( '', ( #6684, #26433 ), #1786 ) ;
#25538=DIRECTION ( 'NONE',  ( -0.8775825618903722036, 0.000000000000000000, 0.4794255386042041156 ) ) ;
#25539=EDGE_CURVE ( 'NONE', #22334, #7778, #25596, .T. ) ;
#25549=DIRECTION ( 'NONE',  ( 0.000000000000000000, -1.000000000000000000, 0.000000000000000000 ) ) ;
#25550=PLANE ( 'NONE',  #16814 ) ;
#25560=AXIS2_PLACEMENT_3D ( 'NONE', #14372, #10390, #14503 ) ;
#25568=DIRECTION ( 'NONE',  ( 0.000000000000000000, 1.000000000000000000, 0.000000000000000000 ) ) ;
#25576=AXIS2_PLACEMENT_3D ( 'NONE', #18391, #16875, #9771 ) ;
#25591=DIRECTION ( 'NONE',  ( -0.4151946956541399669, 0.5000000000001689759, -0.7600087925152558821 ) ) ;
#25596=LINE ( 'NONE', #14086, #13688 ) ;
#25604=DIRECTION ( 'NONE',  ( -0.8775825618903722036, 0.000000000000000000, 0.4794255386042041156 ) ) ;
#25615=AXIS2_PLACEMENT_3D ( 'NONE', #13630, #24862, #4896 ) ;
#25623=ORIENTED_EDGE ( 'NONE', *, *, #14628, .F. ) ;
#25628=DIRECTION ( 'NONE',  ( 0.4794255386042036715, 0.000000000000000000, 0.8775825618903724257 ) ) ;
#25634=TOROIDAL_SURFACE ( 'NONE', #1900, 55.85192378860000417, 0.3499999999999999778 ) ;
#25637=VERTEX_POINT ( 'NONE', #21088 ) ;
#25639=VECTOR ( 'NONE', #13681, 999.9999999999998863 ) ;
#25647=DIRECTION ( 'NONE',  ( 0.000000000000000000, 0.000000000000000000, 1.000000000000000000 ) ) ;
#25664=CARTESIAN_POINT ( 'NONE',  ( 0.000000000000000000, -15.49681045920000066, 0.000000000000000000 ) ) ;
#25669=( LENGTH_UNIT ( ) NAMED_UNIT ( * ) SI_UNIT ( .MILLI., .METRE. ) );
#25677=ORIENTED_EDGE ( 'NONE', *, *, #21253, .T. ) ;
#25681=VECTOR ( 'NONE', #20687, 999.9999999999998863 ) ;
#25685=CARTESIAN_POINT ( 'NONE',  ( 26.69293917519999937, -30.50310889129999836, 48.86109741659999628 ) ) ;
#25687=ORIENTED_EDGE ( 'NONE', *, *, #12420, .T. ) ;
#25733=ORIENTED_EDGE ( 'NONE', *, *, #16324, .T. ) ;
#25736=AXIS2_PLACEMENT_3D ( 'NONE', #24962, #16506, #16639 ) ;
#25737=ORIENTED_EDGE ( 'NONE', *, *, #503, .T. ) ;
#25739=TOROIDAL_SURFACE ( 'NONE', #2491, 19.50000000000000000, 3.000000000000000000 ) ;
#25741=ORIENTED_EDGE ( 'NONE', *, *, #8241, .T. ) ;
#25745=CARTESIAN_POINT ( 'NONE',  ( 5.813199663199999812, -6.776234273679999198, 10.64099060729999913 ) ) ;
#25753=CIRCLE ( 'NONE', #18782, 57.75000000000000000 ) ;
#25767=ADVANCED_FACE ( 'NONE', ( #530 ), #2557, .T. ) ;
#25772=VERTEX_POINT ( 'NONE', #24692 ) ;
#25774=ADVANCED_FACE ( 'NONE', ( #15488 ), #12306, .T. ) ;
#25781=ORIENTED_EDGE ( 'NONE', *, *, #6174, .T. ) ;
#25787=VECTOR ( 'NONE', #24768, 1000.000000000000000 ) ;
#25788=AXIS2_PLACEMENT_3D ( 'NONE', #26962, #25060, #11481 ) ;
#25803=ORIENTED_EDGE ( 'NONE', *, *, #21512, .T. ) ;
#25807=DIRECTION ( 'NONE',  ( 0.000000000000000000, 1.000000000000000000, 0.000000000000000000 ) ) ;
#25808=DIRECTION ( 'NONE',  ( 1.000000000000000000, 0.000000000000000000, 0.000000000000000000 ) ) ;
#25812=TOROIDAL_SURFACE ( 'NONE', #4400, 25.11294200180000047, 0.5000000000000000000 ) ;
#25814=CARTESIAN_POINT ( 'NONE',  ( 3.883346862689999845, -9.250000000000000000, 7.108418751309999450 ) ) ;
#25818=ORIENTED_EDGE ( 'NONE', *, *, #12863, .T. ) ;
#25820=CARTESIAN_POINT ( 'NONE',  ( 0.000000000000000000, -11.55246854740000018, 0.000000000000000000 ) ) ;
#25824=CARTESIAN_POINT ( 'NONE',  ( -26.77683864449999973, -33.79999999999999716, -49.01467436490000296 ) ) ;
#25838=ORIENTED_EDGE ( 'NONE', *, *, #24301, .F. ) ;
#25845=DIRECTION ( 'NONE',  ( 0.000000000000000000, 1.000000000000000000, 0.000000000000000000 ) ) ;
#25871=LINE ( 'NONE', #17114, #3536 ) ;
#25873=CIRCLE ( 'NONE', #4458, 0.3500000000000003664 ) ;
#25877=ORIENTED_EDGE ( 'NONE', *, *, #6204, .T. ) ;
#25881=DIRECTION ( 'NONE',  ( 0.000000000000000000, 0.000000000000000000, 1.000000000000000000 ) ) ;
#25882=EDGE_CURVE ( 'NONE', #6664, #20661, #5315, .T. ) ;
#25887=DIRECTION ( 'NONE',  ( 0.000000000000000000, 1.000000000000000000, 0.000000000000000000 ) ) ;
#25892=DIRECTION ( 'NONE',  ( 1.000000000000000000, 0.000000000000000000, 0.000000000000000000 ) ) ;
#25905=CARTESIAN_POINT ( 'NONE',  ( 0.000000000000000000, -26.59999999999999787, 0.000000000000000000 ) ) ;
#25924=VERTEX_POINT ( 'NONE', #24065 ) ;
#25928=DIRECTION ( 'NONE',  ( 0.4794255386042038936, 0.000000000000000000, 0.8775825618903723147 ) ) ;
#25937=DIRECTION ( 'NONE',  ( 1.000000000000000000, 0.000000000000000000, 0.000000000000000000 ) ) ;
#25942=DIRECTION ( 'NONE',  ( 0.8775825618903722036, 0.000000000000000000, -0.4794255386042041156 ) ) ;
#25949=VERTEX_POINT ( 'NONE', #17373 ) ;
#25954=ORIENTED_EDGE ( 'NONE', *, *, #26851, .T. ) ;
#25959=EDGE_CURVE ( 'NONE', #26635, #8189, #20024, .T. ) ;
#25960=VECTOR ( 'NONE', #17305, 1000.000000000000000 ) ;
#25961=CARTESIAN_POINT ( 'NONE',  ( 9.348798002780000616, -10.50000000000000000, 17.11285995690000306 ) ) ;
#25970=CARTESIAN_POINT ( 'NONE',  ( 26.77683864449999973, -19.40000000000000213, 49.01467436490000296 ) ) ;
#25971=CIRCLE ( 'NONE', #10557, 24.76278252470000041 ) ;
#25974=CARTESIAN_POINT ( 'NONE',  ( -4.500000000000000000, -11.00000000000000000, 40.50000000000000000 ) ) ;
#25987=EDGE_CURVE ( 'NONE', #20862, #10652, #17516, .T. ) ;
#25988=DIRECTION ( 'NONE',  ( 0.4794255386042040046, 0.000000000000000000, 0.8775825618903722036 ) ) ;
#25989=DIRECTION ( 'NONE',  ( 1.000000000000000000, 0.000000000000000000, 0.000000000000000000 ) ) ;
#25994=DIRECTION ( 'NONE',  ( 0.000000000000000000, -1.000000000000000000, 0.000000000000000000 ) ) ;
#25996=LINE ( 'NONE', #12164, #5754 ) ;
#26001=AXIS2_PLACEMENT_3D ( 'NONE', #27830, #7870, #15101 ) ;
#26009=EDGE_CURVE ( 'NONE', #3254, #20039, #26959, .T. ) ;
#26032=DIRECTION ( 'NONE',  ( 0.000000000000000000, 1.000000000000000000, 0.000000000000000000 ) ) ;
#26037=AXIS2_PLACEMENT_3D ( 'NONE', #12007, #12150, #21472 ) ;
#26040=DIRECTION ( 'NONE',  ( 0.000000000000000000, 1.000000000000000000, 0.000000000000000000 ) ) ;
#26042=LINE ( 'NONE', #8254, #9891 ) ;
#26057=ORIENTED_EDGE ( 'NONE', *, *, #1753, .F. ) ;
#26073=CARTESIAN_POINT ( 'NONE',  ( 10.73867332049999845, -11.85850980319999870, 19.65700966069999822 ) ) ;
#26075=DIRECTION ( 'NONE',  ( 0.000000000000000000, 1.000000000000000000, 0.000000000000000000 ) ) ;
#26078=AXIS2_PLACEMENT_3D ( 'NONE', #3981, #17098, #15462 ) ;
#26081=CARTESIAN_POINT ( 'NONE',  ( 26.77683864449999973, -30.20000000000000284, 49.01467436490000296 ) ) ;
#26086=EDGE_LOOP ( 'NONE', ( #15639, #22048, #16058, #5782 ) ) ;
#26093=DIRECTION ( 'NONE',  ( 0.000000000000000000, 1.000000000000000000, 0.000000000000000000 ) ) ;
#26120=AXIS2_PLACEMENT_3D ( 'NONE', #1258, #3152, #19014 ) ;
#26127=CIRCLE ( 'NONE', #4732, 61.35000000000000142 ) ;
#26131=VERTEX_POINT ( 'NONE', #10288 ) ;
#26135=DIRECTION ( 'NONE',  ( 0.4794255386042041156, 0.000000000000000000, 0.8775825618903720926 ) ) ;
#26149=TOROIDAL_SURFACE ( 'NONE', #24268, 55.85192378860000417, 0.3499999999999999778 ) ;
#26151=FACE_OUTER_BOUND ( 'NONE', #22289, .T. ) ;
#26154=CARTESIAN_POINT ( 'NONE',  ( 29.41275679339999982, -37.50000000000000000, 53.83969017199999740 ) ) ;
#26160=EDGE_CURVE ( 'NONE', #28503, #23820, #10147, .T. ) ;
#26162=ORIENTED_EDGE ( 'NONE', *, *, #3612, .F. ) ;
#26168=CYLINDRICAL_SURFACE ( 'NONE', #11113, 57.74999999999999289 ) ;
#26170=LINE ( 'NONE', #26455, #2005 ) ;
#26171=ORIENTED_EDGE ( 'NONE', *, *, #10586, .F. ) ;
#26186=VERTEX_POINT ( 'NONE', #7851 ) ;
#26188=ADVANCED_FACE ( 'NONE', ( #3207 ), #6054, .F. ) ;
#26206=CIRCLE ( 'NONE', #13148, 53.35000000000000142 ) ;
#26209=EDGE_CURVE ( 'NONE', #24400, #54, #19563, .T. ) ;
#26222=FACE_OUTER_BOUND ( 'NONE', #3627, .T. ) ;
#26224=FACE_OUTER_BOUND ( 'NONE', #6155, .T. ) ;
#26225=DIRECTION ( 'NONE',  ( 0.000000000000000000, 1.000000000000000000, 0.000000000000000000 ) ) ;
#26239=ORIENTED_EDGE ( 'NONE', *, *, #19218, .F. ) ;
#26241=ADVANCED_FACE ( 'NONE', ( #24140 ), #25175, .F. ) ;
#26252=DIRECTION ( 'NONE',  ( 0.000000000000000000, 1.000000000000000000, 0.000000000000000000 ) ) ;
#26257=DIRECTION ( 'NONE',  ( 0.000000000000000000, 1.000000000000000000, 0.000000000000000000 ) ) ;
#26261=CARTESIAN_POINT ( 'NONE',  ( -50.00000000000000000, -15.00000000000000000, -2.486899575159999765E-14 ) ) ;
#26278=CARTESIAN_POINT ( 'NONE',  ( 26.69293917519999937, -23.30310889129999907, 48.86109741659999628 ) ) ;
#26287=PRODUCT_DEFINITION ( 'UNKNOWN', '', #20401, #9458 ) ;
#26289=EDGE_CURVE ( 'NONE', #28301, #8830, #19106, .T. ) ;
#26295=ORIENTED_EDGE ( 'NONE', *, *, #13176, .T. ) ;
#26326=ORIENTED_EDGE ( 'NONE', *, *, #10114, .T. ) ;
#26346=PLANE ( 'NONE',  #26664 ) ;
#26356=FACE_OUTER_BOUND ( 'NONE', #28020, .T. ) ;
#26370=DIRECTION ( 'NONE',  ( 0.000000000000000000, 1.000000000000000000, 0.000000000000000000 ) ) ;
#26371=ORIENTED_EDGE ( 'NONE', *, *, #24795, .T. ) ;
#26378=EDGE_CURVE ( 'NONE', #20895, #7380, #11641, .T. ) ;
#26380=DIRECTION ( 'NONE',  ( 1.000000000000000000, 0.000000000000000000, 0.000000000000000000 ) ) ;
#26386=CARTESIAN_POINT ( 'NONE',  ( 28.54979082390000045, -36.85000000000000142, 52.26004156059999417 ) ) ;
#26408=CONICAL_SURFACE ( 'NONE', #21746, 55.67692378859999280, 1.047197551199999799 ) ;
#26410=ORIENTED_EDGE ( 'NONE', *, *, #10370, .F. ) ;
#26433=AXIS2_PLACEMENT_3D ( 'NONE', #27589, #5562, #25255 ) ;
#26447=DIRECTION ( 'NONE',  ( 0.000000000000000000, 1.000000000000000000, 0.000000000000000000 ) ) ;
#26451=EDGE_CURVE ( 'NONE', #5596, #17070, #18662, .T. ) ;
#26455=CARTESIAN_POINT ( 'NONE',  ( 27.68682485439999752, -24.80000000000000071, 50.68039294919999804 ) ) ;
#26464=VECTOR ( 'NONE', #15919, 1000.000000000000114 ) ;
#26466=FACE_BOUND ( 'NONE', #3227, .T. ) ;
#26468=ORIENTED_EDGE ( 'NONE', *, *, #27498, .F. ) ;
#26475=DIRECTION ( 'NONE',  ( 1.000000000000000000, 0.000000000000000000, 0.000000000000000000 ) ) ;
#26479=AXIS2_PLACEMENT_3D ( 'NONE', #28109, #14290, #21000 ) ;
#26480=EDGE_CURVE ( 'NONE', #1234, #12823, #15343, .T. ) ;
#26482=AXIS2_PLACEMENT_3D ( 'NONE', #3155, #21479, #19296 ) ;
#26486=ORIENTED_EDGE ( 'NONE', *, *, #26826, .T. ) ;
#26493=CARTESIAN_POINT ( 'NONE',  ( 31.00000000000000000, -13.00000000000000000, 4.500000000000000000 ) ) ;
#26497=ORIENTED_EDGE ( 'NONE', *, *, #11712, .F. ) ;
#26502=DIRECTION ( 'NONE',  ( 0.000000000000000000, 1.000000000000000000, 0.000000000000000000 ) ) ;
#26506=EDGE_LOOP ( 'NONE', ( #7586, #28654, #16747, #27768 ) ) ;
#26509=DIRECTION ( 'NONE',  ( 0.4794255386042000078, 0.000000000000000000, 0.8775825618903743131 ) ) ;
#26521=ORIENTED_EDGE ( 'NONE', *, *, #20226, .F. ) ;
#26531=ORIENTED_EDGE ( 'NONE', *, *, #1186, .T. ) ;
#26542=AXIS2_PLACEMENT_3D ( 'NONE', #19291, #6158, #26135 ) ;
#26544=VECTOR ( 'NONE', #12067, 999.9999999999998863 ) ;
#26557=CARTESIAN_POINT ( 'NONE',  ( 27.68682485439999752, -35.29999999999999716, 50.68039294919999804 ) ) ;
#26560=DIRECTION ( 'NONE',  ( 0.000000000000000000, 1.000000000000000000, 0.000000000000000000 ) ) ;
#26561=AXIS2_PLACEMENT_3D ( 'NONE', #14, #6557, #26665 ) ;
#26565=EDGE_LOOP ( 'NONE', ( #11524, #27575, #7252, #24480 ) ) ;
#26575=DIRECTION ( 'NONE',  ( 1.000000000000000000, 0.000000000000000000, 0.000000000000000000 ) ) ;
#26578=CARTESIAN_POINT ( 'NONE',  ( 0.000000000000000000, -39.32601556110000018, 0.000000000000000000 ) ) ;
#26583=CARTESIAN_POINT ( 'NONE',  ( -4.500000000000000000, 0.000000000000000000, 31.00000000000000000 ) ) ;
#26587=VECTOR ( 'NONE', #23614, 999.9999999999998863 ) ;
#26602=TOROIDAL_SURFACE ( 'NONE', #21488, 55.85192378860000417, 0.3499999999999999778 ) ;
#26606=EDGE_CURVE ( 'NONE', #2986, #28714, #22862, .T. ) ;
#26608=DIRECTION ( 'NONE',  ( 0.000000000000000000, 1.000000000000000000, 0.000000000000000000 ) ) ;
#26631=DIRECTION ( 'NONE',  ( 0.4794255386042041156, 0.000000000000000000, 0.8775825618903719816 ) ) ;
#26635=VERTEX_POINT ( 'NONE', #13891 ) ;
#26664=AXIS2_PLACEMENT_3D ( 'NONE', #2464, #12909, #10719 ) ;
#26665=DIRECTION ( 'NONE',  ( 1.000000000000000000, 0.000000000000000000, 0.000000000000000000 ) ) ;
#26690=ORIENTED_EDGE ( 'NONE', *, *, #3244, .T. ) ;
#26696=EDGE_CURVE ( 'NONE', #28503, #20661, #10070, .T. ) ;
#26705=CIRCLE ( 'NONE', #20663, 9.500000000000001776 ) ;
#26718=DIRECTION ( 'NONE',  ( 1.000000000000000000, 0.000000000000000000, 0.000000000000000000 ) ) ;
#26731=VERTEX_POINT ( 'NONE', #11984 ) ;
#26735=EDGE_CURVE ( 'NONE', #77, #28180, #21308, .T. ) ;
#26751=CIRCLE ( 'NONE', #6738, 2.999999999999998224 ) ;
#26764=DIRECTION ( 'NONE',  ( 0.4794255386042036715, 0.000000000000000000, 0.8775825618903724257 ) ) ;
#26765=DIRECTION ( 'NONE',  ( 0.4794255386042041156, 0.000000000000000000, 0.8775825618903722036 ) ) ;
#26768=CARTESIAN_POINT ( 'NONE',  ( 29.41275679339999982, -25.00000000000000000, 53.83969017199999740 ) ) ;
#26782=ORIENTED_EDGE ( 'NONE', *, *, #28067, .F. ) ;
#26784=CIRCLE ( 'NONE', #3526, 57.75000000000000000 ) ;
#26806=DIRECTION ( 'NONE',  ( 0.000000000000000000, 1.000000000000000000, 0.000000000000000000 ) ) ;
#26809=VERTEX_POINT ( 'NONE', #28695 ) ;
#26815=AXIS2_PLACEMENT_3D ( 'NONE', #9632, #7761, #14304 ) ;
#26817=DIRECTION ( 'NONE',  ( 1.000000000000000000, 0.000000000000000000, 0.000000000000000000 ) ) ;
#26821=CARTESIAN_POINT ( 'NONE',  ( 26.69293917519999937, -15.49689110870000164, 48.86109741659999628 ) ) ;
#26826=EDGE_CURVE ( 'NONE', #4674, #22328, #20545, .T. ) ;
#26828=CARTESIAN_POINT ( 'NONE',  ( -26.60903970598167589, -33.79999999999999716, -48.70752046822583736 ) ) ;
#26836=ORIENTED_EDGE ( 'NONE', *, *, #2528, .F. ) ;
#26837=CARTESIAN_POINT ( 'NONE',  ( 0.000000000000000000, -39.50000000000000000, 0.000000000000000000 ) ) ;
#26843=LINE ( 'NONE', #22619, #14516 ) ;
#26851=EDGE_CURVE ( 'NONE', #10652, #19426, #64, .T. ) ;
#26854=DIRECTION ( 'NONE',  ( 0.000000000000000000, 1.000000000000000000, 0.000000000000000000 ) ) ;
#26858=EDGE_CURVE ( 'NONE', #15395, #13005, #24647, .T. ) ;
#26882=ORIENTED_EDGE ( 'NONE', *, *, #27087, .T. ) ;
#26886=EDGE_CURVE ( 'NONE', #1234, #1856, #15594, .T. ) ;
#26891=CARTESIAN_POINT ( 'NONE',  ( 0.000000000000000000, -2.000000000000000000, 0.000000000000000000 ) ) ;
#26908=DIRECTION ( 'NONE',  ( 0.000000000000000000, 1.000000000000000000, 0.000000000000000000 ) ) ;
#26909=DIRECTION ( 'NONE',  ( 0.000000000000000000, 1.000000000000000000, 0.000000000000000000 ) ) ;
#26921=CARTESIAN_POINT ( 'NONE',  ( 0.000000000000000000, -33.49689110869999809, 0.000000000000000000 ) ) ;
#26941=ORIENTED_EDGE ( 'NONE', *, *, #6518, .F. ) ;
#26949=CIRCLE ( 'NONE', #4129, 52.35000000000000142 ) ;
#26953=ORIENTED_EDGE ( 'NONE', *, *, #18989, .T. ) ;
#26954=CIRCLE ( 'NONE', #26479, 0.9999999999999980016 ) ;
#26959=LINE ( 'NONE', #16151, #14465 ) ;
#26962=CARTESIAN_POINT ( 'NONE',  ( 0.000000000000000000, -2.000000000000000000, 0.000000000000000000 ) ) ;
#26969=CARTESIAN_POINT ( 'NONE',  ( -27.68147801010000109, -38.34400911419999858, -50.67060561630000137 ) ) ;
#26970=CONICAL_SURFACE ( 'NONE', #739, 55.67692378859999280, 1.047197551199999799 ) ;
#26972=CARTESIAN_POINT ( 'NONE',  ( 0.000000000000000000, -13.50000000000000000, 0.000000000000000000 ) ) ;
#26973=CARTESIAN_POINT ( 'NONE',  ( 0.000000000000000000, -16.00000000000000000, 0.000000000000000000 ) ) ;
#26975=CARTESIAN_POINT ( 'NONE',  ( 50.00000000000000000, -11.00000000000000000, 4.500000000000000000 ) ) ;
#26988=DIRECTION ( 'NONE',  ( 0.000000000000000000, 1.000000000000000000, 0.000000000000000000 ) ) ;
#26990=VERTEX_POINT ( 'NONE', #25511 ) ;
#26996=EDGE_CURVE ( 'NONE', #23820, #7778, #2384, .T. ) ;
#26997=FACE_OUTER_BOUND ( 'NONE', #3321, .T. ) ;
#27012=TOROIDAL_SURFACE ( 'NONE', #8836, 19.50000000000000000, 7.000000000000000000 ) ;
#27020=CARTESIAN_POINT ( 'NONE',  ( 0.000000000000000000, -2.000000000000000000, 0.000000000000000000 ) ) ;
#27031=EDGE_CURVE ( 'NONE', #4012, #2845, #3764, .T. ) ;
#27034=VECTOR ( 'NONE', #23340, 1000.000000000000000 ) ;
#27051=AXIS2_PLACEMENT_3D ( 'NONE', #20457, #22509, #11402 ) ;
#27054=AXIS2_PLACEMENT_3D ( 'NONE', #5906, #3734, #19324 ) ;
#27069=FACE_OUTER_BOUND ( 'NONE', #6503, .T. ) ;
#27081=LINE ( 'NONE', #23140, #9433 ) ;
#27087=EDGE_CURVE ( 'NONE', #8439, #18617, #21016, .T. ) ;
#27095=LINE ( 'NONE', #20826, #25681 ) ;
#27101=ORIENTED_EDGE ( 'NONE', *, *, #26378, .T. ) ;
#27102=CARTESIAN_POINT ( 'NONE',  ( -1.598721155459999804E-14, -11.00000000000000000, 50.00000000000000000 ) ) ;
#27104=DIRECTION ( 'NONE',  ( 0.000000000000000000, 1.000000000000000000, 0.000000000000000000 ) ) ;
#27135=FACE_OUTER_BOUND ( 'NONE', #18560, .T. ) ;
#27138=VECTOR ( 'NONE', #23521, 1000.000000000000000 ) ;
#27152=ORIENTED_EDGE ( 'NONE', *, *, #669, .F. ) ;
#27170=AXIS2_PLACEMENT_3D ( 'NONE', #22065, #17253, #76 ) ;
#27179=CIRCLE ( 'NONE', #9485, 9.499999999999998224 ) ;
#27196=ADVANCED_FACE ( 'NONE', ( #22149 ), #7048, .T. ) ;
#27199=DIRECTION ( 'NONE',  ( 0.8775825618903722036, 0.000000000000000000, -0.4794255386042041156 ) ) ;
#27205=AXIS2_PLACEMENT_3D ( 'NONE', #11597, #9419, #20505 ) ;
#27210=DIRECTION ( 'NONE',  ( 1.000000000000000000, 0.000000000000000000, 0.000000000000000000 ) ) ;
#27211=VERTEX_POINT ( 'NONE', #20103 ) ;
#27214=ORIENTED_EDGE ( 'NONE', *, *, #2417, .T. ) ;
#27215=DIRECTION ( 'NONE',  ( 1.000000000000000000, 0.000000000000000000, 0.000000000000000000 ) ) ;
#27218=ORIENTED_EDGE ( 'NONE', *, *, #16888, .F. ) ;
#27227=DIRECTION ( 'NONE',  ( 0.4794255386042036715, 0.000000000000000000, 0.8775825618903724257 ) ) ;
#27231=AXIS2_PLACEMENT_3D ( 'NONE', #12244, #16623, #21156 ) ;
#27233=DIRECTION ( 'NONE',  ( 0.000000000000000000, 1.000000000000000000, 0.000000000000000000 ) ) ;
#27242=ORIENTED_EDGE ( 'NONE', *, *, #11749, .F. ) ;
#27244=CIRCLE ( 'NONE', #4411, 1.999999999999999556 ) ;
#27249=EDGE_LOOP ( 'NONE', ( #25494, #14817, #7309, #2573 ) ) ;
#27253=EDGE_CURVE ( 'NONE', #14280, #25949, #26127, .T. ) ;
#27280=CARTESIAN_POINT ( 'NONE',  ( 0.000000000000000000, -10.50000000000000000, 0.000000000000000000 ) ) ;
#27285=DIRECTION ( 'NONE',  ( 1.000000000000000000, 0.000000000000000000, 0.000000000000000000 ) ) ;
#27288=DIRECTION ( 'NONE',  ( 0.4794255386042040046, 0.000000000000000000, 0.8775825618903722036 ) ) ;
#27291=EDGE_CURVE ( 'NONE', #17070, #2258, #21035, .T. ) ;
#27339=CARTESIAN_POINT ( 'NONE',  ( 0.000000000000000000, -37.08699221940000257, 0.000000000000000000 ) ) ;
#27350=DIRECTION ( 'NONE',  ( 0.4794255386042040046, 0.000000000000000000, 0.8775825618903722036 ) ) ;
#27353=ORIENTED_EDGE ( 'NONE', *, *, #12697, .F. ) ;
#27354=EDGE_CURVE ( 'NONE', #11126, #11154, #3793, .T. ) ;
#27358=EDGE_CURVE ( 'NONE', #13005, #20039, #6103, .T. ) ;
#27369=CARTESIAN_POINT ( 'NONE',  ( -27.18988201479999844, -22.09844555429999957, -49.77074518290000071 ) ) ;
#27371=ORIENTED_EDGE ( 'NONE', *, *, #13175, .T. ) ;
#27375=CIRCLE ( 'NONE', #6902, 55.67692378859999991 ) ;
#27378=ORIENTED_EDGE ( 'NONE', *, *, #28515, .F. ) ;
#27419=CIRCLE ( 'NONE', #2280, 55.50192378860000275 ) ;
#27422=ORIENTED_EDGE ( 'NONE', *, *, #17008, .F. ) ;
#27436=EDGE_CURVE ( 'NONE', #18033, #5395, #5195, .T. ) ;
#27437=CARTESIAN_POINT ( 'NONE',  ( -28.07036528529999941, -39.41300778060000454, -51.38245899869999533 ) ) ;
#27443=AXIS2_PLACEMENT_3D ( 'NONE', #14434, #23597, #27978 ) ;
#27446=ORIENTED_EDGE ( 'NONE', *, *, #2781, .T. ) ;
#27448=CARTESIAN_POINT ( 'NONE',  ( 26.77683864449999973, -23.00000000000000000, 49.01467436490000296 ) ) ;
#27468=DIRECTION ( 'NONE',  ( 0.000000000000000000, 0.000000000000000000, 1.000000000000000000 ) ) ;
#27473=ORIENTED_EDGE ( 'NONE', *, *, #15189, .F. ) ;
#27478=CYLINDRICAL_SURFACE ( 'NONE', #25257, 57.74999999999999289 ) ;
#27480=AXIS2_PLACEMENT_3D ( 'NONE', #5485, #18755, #22984 ) ;
#27498=EDGE_CURVE ( 'NONE', #1871, #26731, #11139, .T. ) ;
#27502=DIRECTION ( 'NONE',  ( 0.4794255386042040601, 0.000000000000000000, 0.8775825618903720926 ) ) ;
#27509=AXIS2_PLACEMENT_3D ( 'NONE', #8923, #15042, #13441 ) ;
#27522=EDGE_LOOP ( 'NONE', ( #16591, #4480, #15544, #11936 ) ) ;
#27524=DIRECTION ( 'NONE',  ( 0.4151946956541399669, 0.5000000000001689759, 0.7600087925152558821 ) ) ;
#27525=FACE_OUTER_BOUND ( 'NONE', #24105, .T. ) ;
#27527=VECTOR ( 'NONE', #14004, 1000.000000000000114 ) ;
#27532=CARTESIAN_POINT ( 'NONE',  ( 27.18988201479999844, -22.09844555429999957, 49.77074518290000071 ) ) ;
#27544=CARTESIAN_POINT ( 'NONE',  ( 27.18988201479999844, -16.70155444569999759, 49.77074518290000071 ) ) ;
#27554=CARTESIAN_POINT ( 'NONE',  ( 40.50000000000000000, -11.00000000000000000, -4.500000000000000000 ) ) ;
#27556=ORIENTED_EDGE ( 'NONE', *, *, #1746, .F. ) ;
#27561=EDGE_LOOP ( 'NONE', ( #3195, #13262, #8732, #16478 ) ) ;
#27571=ADVANCED_FACE ( 'NONE', ( #20654 ), #6034, .F. ) ;
#27575=ORIENTED_EDGE ( 'NONE', *, *, #27358, .T. ) ;
#27584=DIRECTION ( 'NONE',  ( 0.4794255386042040046, 0.000000000000000000, 0.8775825618903722036 ) ) ;
#27589=CARTESIAN_POINT ( 'NONE',  ( 0.000000000000000000, 0.000000000000000000, 0.000000000000000000 ) ) ;
#27596=DIRECTION ( 'NONE',  ( 1.000000000000000000, 0.000000000000000000, 0.000000000000000000 ) ) ;
#27597=EDGE_LOOP ( 'NONE', ( #2599, #17476 ) ) ;
#27605=EDGE_LOOP ( 'NONE', ( #9076, #128, #16710, #1454 ) ) ;
#27612=CIRCLE ( 'NONE', #18760, 0.3500000000000003664 ) ;
#27613=CARTESIAN_POINT ( 'NONE',  ( 0.000000000000000000, -10.50000000000000000, 0.000000000000000000 ) ) ;
#27625=CIRCLE ( 'NONE', #14995, 57.75000000000000000 ) ;
#27634=SURFACE_SIDE_STYLE ('',( #14066 ) ) ;
#27649=DIRECTION ( 'NONE',  ( 0.000000000000000000, -1.000000000000000000, 0.000000000000000000 ) ) ;
#27657=ORIENTED_EDGE ( 'NONE', *, *, #25539, .F. ) ;
#27660=AXIS2_PLACEMENT_3D ( 'NONE', #3442, #3994, #1269 ) ;
#27672=DIRECTION ( 'NONE',  ( 0.000000000000000000, 1.000000000000000000, 0.000000000000000000 ) ) ;
#27681=AXIS2_PLACEMENT_3D ( 'NONE', #15509, #4456, #26764 ) ;
#27687=CARTESIAN_POINT ( 'NONE',  ( 0.000000000000000000, -30.20000000000000284, 0.000000000000000000 ) ) ;
#27691=ORIENTED_EDGE ( 'NONE', *, *, #17570, .T. ) ;
#27702=EDGE_LOOP ( 'NONE', ( #23572, #23720, #8808, #13774 ) ) ;
#27712=FACE_OUTER_BOUND ( 'NONE', #509, .T. ) ;
#27713=CARTESIAN_POINT ( 'NONE',  ( 0.000000000000000000, -33.79999999999999716, 0.000000000000000000 ) ) ;
#27719=CONICAL_SURFACE ( 'NONE', #16471, 52.86371681419998936, 1.437659999240000097 ) ;
#27723=DIRECTION ( 'NONE',  ( 1.000000000000000000, 0.000000000000000000, 0.000000000000000000 ) ) ;
#27732=EDGE_LOOP ( 'NONE', ( #190, #25308, #1757, #14358 ) ) ;
#27734=DIRECTION ( 'NONE',  ( -0.000000000000000000, 1.000000000000000000, 0.000000000000000000 ) ) ;
#27764=( NAMED_UNIT ( * ) PLANE_ANGLE_UNIT ( ) SI_UNIT ( $, .RADIAN. ) );
#27768=ORIENTED_EDGE ( 'NONE', *, *, #26886, .F. ) ;
#27775=DIRECTION ( 'NONE',  ( 0.4794255386042000078, 0.000000000000000000, 0.8775825618903743131 ) ) ;
#27785=ADVANCED_FACE ( 'NONE', ( #20307 ), #13847, .T. ) ;
#27787=DIRECTION ( 'NONE',  ( 0.4794255386042000078, 0.000000000000000000, 0.8775825618903743131 ) ) ;
#27790=CARTESIAN_POINT ( 'NONE',  ( 50.00000000000000000, -15.00000000000000000, -4.500000000000000000 ) ) ;
#27797=EDGE_LOOP ( 'NONE', ( #16020, #13051, #12992, #19354 ) ) ;
#27806=PLANE ( 'NONE',  #4750 ) ;
#27813=CARTESIAN_POINT ( 'NONE',  ( 31.00000000000000000, -11.00000000000000000, -4.500000000000000000 ) ) ;
#27821=VECTOR ( 'NONE', #28094, 1000.000000000000114 ) ;
#27830=CARTESIAN_POINT ( 'NONE',  ( -25.09792694589999940, -16.00000000000000000, -45.94144711499999545 ) ) ;
#27844=FACE_OUTER_BOUND ( 'NONE', #1595, .T. ) ;
#27846=CARTESIAN_POINT ( 'NONE',  ( -26.69293917519999937, -19.70310889130000120, -48.86109741659999628 ) ) ;
#27855=EDGE_CURVE ( 'NONE', #2986, #13987, #3279, .T. ) ;
#27860=DIRECTION ( 'NONE',  ( 0.000000000000000000, 1.000000000000000000, 0.000000000000000000 ) ) ;
#27863=EDGE_CURVE ( 'NONE', #12535, #584, #2223, .T. ) ;
#27880=ORIENTED_EDGE ( 'NONE', *, *, #19891, .T. ) ;
#27881=CONICAL_SURFACE ( 'NONE', #385, 55.67692378859999280, 1.047197551199999799 ) ;
#27882=AXIS2_PLACEMENT_3D ( 'NONE', #25961, #23770, #3813 ) ;
#27885=CIRCLE ( 'NONE', #19044, 0.4999999999999990008 ) ;
#27890=CARTESIAN_POINT ( 'NONE',  ( -4.500000000000000000, -15.00000000000000000, -50.00000000000000000 ) ) ;
#27891=DIRECTION ( 'NONE',  ( 0.000000000000000000, -1.000000000000000000, 0.000000000000000000 ) ) ;
#27894=ORIENTED_EDGE ( 'NONE', *, *, #6243, .F. ) ;
#27902=CIRCLE ( 'NONE', #19066, 60.85000000000000142 ) ;
#27913=LINE ( 'NONE', #14906, #11826 ) ;
#27923=AXIS2_PLACEMENT_3D ( 'NONE', #12186, #11902, #18771 ) ;
#27930=DIRECTION ( 'NONE',  ( 0.000000000000000000, 1.000000000000000000, 0.000000000000000000 ) ) ;
#27931=VERTEX_POINT ( 'NONE', #16660 ) ;
#27960=AXIS2_PLACEMENT_3D ( 'NONE', #7616, #5411, #16758 ) ;
#27966=CARTESIAN_POINT ( 'NONE',  ( -26.60903970598167589, -15.80000000000000071, -48.70752046822583736 ) ) ;
#27971=CARTESIAN_POINT ( 'NONE',  ( -26.69293917519999937, -26.29689110869999880, -48.86109741659999628 ) ) ;
#27978=DIRECTION ( 'NONE',  ( 1.000000000000000000, 0.000000000000000000, 0.000000000000000000 ) ) ;
#27993=EDGE_CURVE ( 'NONE', #26731, #20895, #6862, .T. ) ;
#27996=AXIS2_PLACEMENT_3D ( 'NONE', #16827, #14630, #23529 ) ;
#27998=FACE_OUTER_BOUND ( 'NONE', #12317, .T. ) ;
#28004=DIRECTION ( 'NONE',  ( 1.000000000000000000, 0.000000000000000000, 0.000000000000000000 ) ) ;
#28008=FACE_OUTER_BOUND ( 'NONE', #27561, .T. ) ;
#28014=ORIENTED_EDGE ( 'NONE', *, *, #14543, .F. ) ;
#28020=EDGE_LOOP ( 'NONE', ( #25305, #22552, #20770, #5910 ) ) ;
#28039=ORIENTED_EDGE ( 'NONE', *, *, #11974, .F. ) ;
#28040=STYLED_ITEM ( 'NONE', ( #16542 ), #6684 ) ;
#28044=AXIS2_PLACEMENT_3D ( 'NONE', #18547, #4987, #20589 ) ;
#28055=FACE_OUTER_BOUND ( 'NONE', #24767, .T. ) ;
#28067=EDGE_CURVE ( 'NONE', #12325, #6364, #1742, .T. ) ;
#28089=CARTESIAN_POINT ( 'NONE',  ( 11.69905354509999995, -15.49681045920000066, 21.41497386989999896 ) ) ;
#28094=DIRECTION ( 'NONE',  ( 0.4381045938801422235, -0.4061384660531317525, 0.8019450799232605842 ) ) ;
#28098=ORIENTED_EDGE ( 'NONE', *, *, #12276, .F. ) ;
#28109=CARTESIAN_POINT ( 'NONE',  ( -27.59093974670000193, -39.32601556110000018, -50.50487643680000360 ) ) ;
#28111=VERTEX_POINT ( 'NONE', #10182 ) ;
#28121=DIRECTION ( 'NONE',  ( 0.000000000000000000, 1.000000000000000000, 0.000000000000000000 ) ) ;
#28123=CARTESIAN_POINT ( 'NONE',  ( 0.000000000000000000, -10.95575221240000019, 0.000000000000000000 ) ) ;
#28125=DIRECTION ( 'NONE',  ( 0.000000000000000000, 1.000000000000000000, 0.000000000000000000 ) ) ;
#28131=ADVANCED_FACE ( 'NONE', ( #5960 ), #26408, .T. ) ;
#28132=EDGE_LOOP ( 'NONE', ( #7882, #15934, #17720, #9123 ) ) ;
#28133=CARTESIAN_POINT ( 'NONE',  ( 28.44874375979999925, -10.08849557519999962, 52.07507615039999394 ) ) ;
#28136=CARTESIAN_POINT ( 'NONE',  ( 0.000000000000000000, -26.59999999999999787, 0.000000000000000000 ) ) ;
#28137=ORIENTED_EDGE ( 'NONE', *, *, #23275, .F. ) ;
#28164=ORIENTED_EDGE ( 'NONE', *, *, #17902, .F. ) ;
#28165=EDGE_CURVE ( 'NONE', #1181, #25772, #9171, .T. ) ;
#28170=DIRECTION ( 'NONE',  ( 0.4794255386042042266, 0.000000000000000000, 0.8775825618903720926 ) ) ;
#28172=EDGE_LOOP ( 'NONE', ( #2195, #10310, #25877, #12647 ) ) ;
#28180=VERTEX_POINT ( 'NONE', #26073 ) ;
#28182=EDGE_CURVE ( 'NONE', #8439, #4998, #28251, .T. ) ;
#28197=CARTESIAN_POINT ( 'NONE',  ( 4.500000000000000000, -11.00000000000000000, -31.00000000000000000 ) ) ;
#28212=ORIENTED_EDGE ( 'NONE', *, *, #18470, .T. ) ;
#28219=ADVANCED_FACE ( 'NONE', ( #7888 ), #23163, .T. ) ;
#28231=ORIENTED_EDGE ( 'NONE', *, *, #12697, .T. ) ;
#28236=CIRCLE ( 'NONE', #12428, 19.50000000000000000 ) ;
#28244=CARTESIAN_POINT ( 'NONE',  ( 26.69293917519999937, -26.29689110869999880, 48.86109741659999628 ) ) ;
#28249=ADVANCED_FACE ( 'NONE', ( #1212 ), #4545, .T. ) ;
#28251=LINE ( 'NONE', #3794, #8236 ) ;
#28258=LINE ( 'NONE', #4071, #26587 ) ;
#28279=EDGE_LOOP ( 'NONE', ( #18519, #3871, #3071, #17896 ) ) ;
#28280=AXIS2_PLACEMENT_3D ( 'NONE', #8567, #23883, #6093 ) ;
#28284=DIRECTION ( 'NONE',  ( 0.000000000000000000, 0.000000000000000000, -1.000000000000000000 ) ) ;
#28293=ORIENTED_EDGE ( 'NONE', *, *, #7668, .T. ) ;
#28297=AXIS2_PLACEMENT_3D ( 'NONE', #20090, #15402, #24316 ) ;
#28301=VERTEX_POINT ( 'NONE', #17046 ) ;
#28317=VECTOR ( 'NONE', #19265, 1000.000000000000000 ) ;
#28320=CYLINDRICAL_SURFACE ( 'NONE', #17281, 57.74999999999999289 ) ;
#28324=AXIS2_PLACEMENT_3D ( 'NONE', #17207, #10478, #2068 ) ;
#28329=CARTESIAN_POINT ( 'NONE',  ( 0.000000000000000000, -15.00000000000000000, 52.35000000000000142 ) ) ;
#28341=AXIS2_PLACEMENT_3D ( 'NONE', #26837, #9328, #11362 ) ;
#28346=ORIENTED_EDGE ( 'NONE', *, *, #20275, .T. ) ;
#28348=ADVANCED_FACE ( 'NONE', ( #26224 ), #12893, .T. ) ;
#28353=ORIENTED_EDGE ( 'NONE', *, *, #26480, .F. ) ;
#28359=VECTOR ( 'NONE', #5162, 999.9999999999998863 ) ;
#28370=VERTEX_POINT ( 'NONE', #13085 ) ;
#28379=TOROIDAL_SURFACE ( 'NONE', #19084, 55.85192378860000417, 0.3499999999999999778 ) ;
#28393=DIRECTION ( 'NONE',  ( 0.000000000000000000, 1.000000000000000000, 0.000000000000000000 ) ) ;
#28401=ORIENTED_EDGE ( 'NONE', *, *, #25959, .F. ) ;
#28405=DIRECTION ( 'NONE',  ( 1.000000000000000000, 0.000000000000000000, 0.000000000000000000 ) ) ;
#28409=ADVANCED_FACE ( 'NONE', ( #8705 ), #6889, .F. ) ;
#28412=CARTESIAN_POINT ( 'NONE',  ( 0.000000000000000000, -16.50000000000000000, 0.000000000000000000 ) ) ;
#28419=AXIS2_PLACEMENT_3D ( 'NONE', #6331, #26447, #23681 ) ;
#28460=AXIS2_PLACEMENT_3D ( 'NONE', #28630, #22092, #4454 ) ;
#28472=FACE_BOUND ( 'NONE', #21175, .T. ) ;
#28476=ADVANCED_FACE ( 'NONE', ( #11783 ), #9683, .F. ) ;
#28479=AXIS2_PLACEMENT_3D ( 'NONE', #10100, #19671, #24045 ) ;
#28482=DIRECTION ( 'NONE',  ( 0.000000000000000000, 1.000000000000000000, 0.000000000000000000 ) ) ;
#28483=AXIS2_PLACEMENT_3D ( 'NONE', #10369, #19285, #28170 ) ;
#28503=VERTEX_POINT ( 'NONE', #459 ) ;
#28510=CONICAL_SURFACE ( 'NONE', #6177, 55.67692378859999280, 1.047197551199999799 ) ;
#28515=EDGE_CURVE ( 'NONE', #4628, #21477, #20856, .T. ) ;
#28522=VECTOR ( 'NONE', #9137, 1000.000000000000000 ) ;
#28524=DIRECTION ( 'NONE',  ( 0.000000000000000000, 1.000000000000000000, 0.000000000000000000 ) ) ;
#28533=DIRECTION ( 'NONE',  ( 0.000000000000000000, 1.000000000000000000, 0.000000000000000000 ) ) ;
#28534=TOROIDAL_SURFACE ( 'NONE', #7162, 55.85192378860000417, 0.3499999999999999778 ) ;
#28538=DIRECTION ( 'NONE',  ( -0.3422283636740854340, -0.7003189540771749266, -0.6264448177271558782 ) ) ;
#28544=CIRCLE ( 'NONE', #11343, 57.75000000000000000 ) ;
#28547=EDGE_LOOP ( 'NONE', ( #1654, #15875, #19554, #2887 ) ) ;
#28553=DIRECTION ( 'NONE',  ( 1.000000000000000000, 0.000000000000000000, 0.000000000000000000 ) ) ;
#28569=ORIENTED_EDGE ( 'NONE', *, *, #13926, .F. ) ;
#28612=AXIS2_PLACEMENT_3D ( 'NONE', #19836, #1945, #4260 ) ;
#28613=DIRECTION ( 'NONE',  ( 0.000000000000000000, -1.000000000000000000, 0.000000000000000000 ) ) ;
#28614=DIRECTION ( 'NONE',  ( 1.000000000000000000, 0.000000000000000000, 0.000000000000000000 ) ) ;
#28630=CARTESIAN_POINT ( 'NONE',  ( 0.000000000000000000, -22.69689110870000093, 0.000000000000000000 ) ) ;
#28633=AXIS2_PLACEMENT_3D ( 'NONE', #18398, #24950, #11962 ) ;
#28639=CARTESIAN_POINT ( 'NONE',  ( -27.68682485439999752, -36.20000000000000284, -50.68039294919999804 ) ) ;
#28647=CARTESIAN_POINT ( 'NONE',  ( 0.000000000000000000, -17.89999999999999858, 0.000000000000000000 ) ) ;
#28653=CARTESIAN_POINT ( 'NONE',  ( -27.68682485439999752, -24.50000000000000000, -50.68039294919999804 ) ) ;
#28654=ORIENTED_EDGE ( 'NONE', *, *, #25218, .T. ) ;
#28665=CARTESIAN_POINT ( 'NONE',  ( -9.348798002780000616, -10.50000000000000000, -17.11285995690000306 ) ) ;
#28682=ORIENTED_EDGE ( 'NONE', *, *, #27031, .T. ) ;
#28695=CARTESIAN_POINT ( 'NONE',  ( -50.00000000000000000, -11.00000000000000000, -4.500000000000000000 ) ) ;
#28703=AXIS2_PLACEMENT_3D ( 'NONE', #16829, #5184, #23110 ) ;
#28714=VERTEX_POINT ( 'NONE', #13128 ) ;
#28719=ORIENTED_EDGE ( 'NONE', *, *, #2371, .T. ) ;
#28731=EDGE_CURVE ( 'NONE', #13393, #26990, #25971, .T. ) ;
#28737=CARTESIAN_POINT ( 'NONE',  ( 0.000000000000000000, -22.69689110870000093, 0.000000000000000000 ) ) ;
#28743=DIRECTION ( 'NONE',  ( 0.000000000000000000, 1.000000000000000000, 0.000000000000000000 ) ) ;
#28763=ORIENTED_EDGE ( 'NONE', *, *, #1222, .F. ) ;
#28780=DIRECTION ( 'NONE',  ( -0.8775825618903722036, 0.000000000000000000, 0.4794255386042041156 ) ) ;
#28785=VECTOR ( 'NONE', #25549, 1000.000000000000000 ) ;
ENDSEC;
END-ISO-10303-21;
